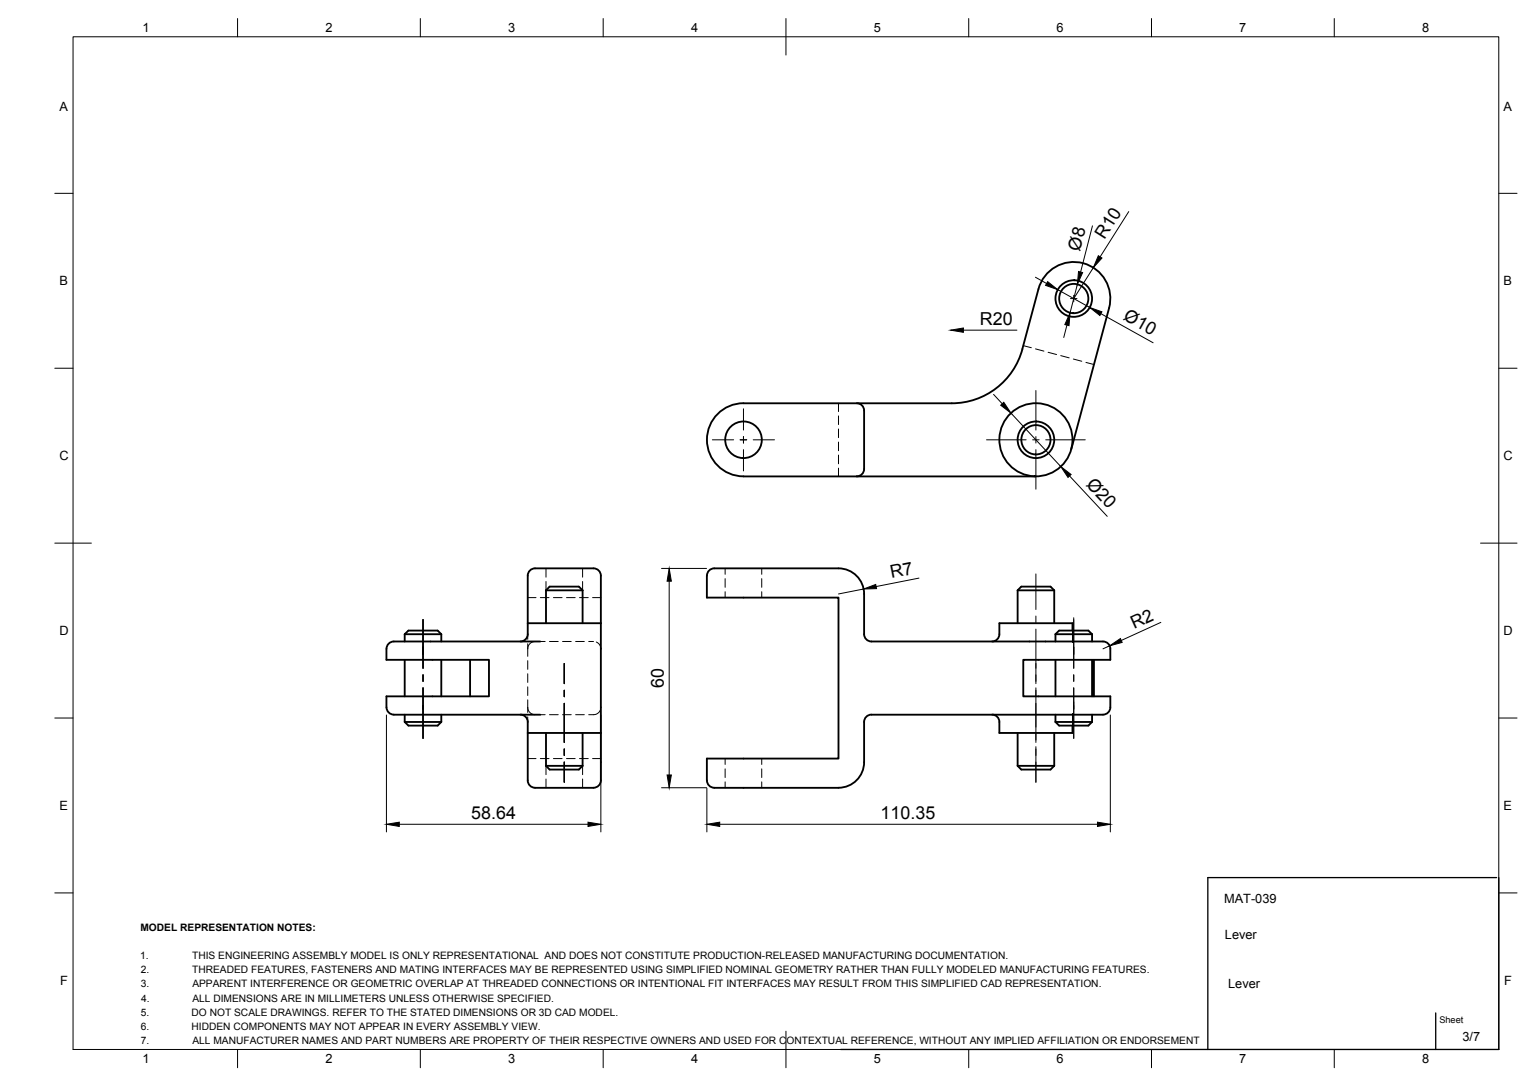
ISO-10303-21;
HEADER;
/* Generated by software containing ST-Developer
 * from STEP Tools, Inc. (www.steptools.com) 
 */

FILE_DESCRIPTION(
/* description */ ('STEP AP214'),
/* implementation_level */ '2;1');

FILE_NAME(
/* name */ 'Lever.step',
/* time_stamp */ '2026-11-14T21:46:24-08:00',
/* author */ (''),
/* organization */ (''),
/* preprocessor_version */ 'ST-DEVELOPER v20.2',
/* originating_system */ 'Autodesk Translation Framework v15.17.0.0',
/* authorisation */ '');

FILE_SCHEMA (('AUTOMOTIVE_DESIGN { 1 0 10303 214 3 1 1 }'));
ENDSEC;

DATA;
#10=MECHANICAL_DESIGN_GEOMETRIC_PRESENTATION_REPRESENTATION('',(#93),#7783);
#11=(
BOUNDED_SURFACE()
B_SPLINE_SURFACE(3,2,((#7242,#7243,#7244),(#7245,#7246,#7247),(#7248,#7249,
#7250),(#7251,#7252,#7253),(#7254,#7255,#7256),(#7257,#7258,#7259),(#7260,
#7261,#7262),(#7263,#7264,#7265),(#7266,#7267,#7268),(#7269,#7270,#7271),
(#7272,#7273,#7274),(#7275,#7276,#7277),(#7278,#7279,#7280),(#7281,#7282,
#7283)),.UNSPECIFIED.,.F.,.F.,.F.)
B_SPLINE_SURFACE_WITH_KNOTS((4,2,2,2,2,2,4),(3,3),(0.00201286221565559,
0.00340012561105001,0.00476544226438698,0.00613075891772395,0.00749607557106092,
0.0102267088777349,0.0129573421844088),(0.,1.00002194674206),
 .UNSPECIFIED.)
GEOMETRIC_REPRESENTATION_ITEM()
RATIONAL_B_SPLINE_SURFACE(((1.,0.706119316799645,1.0000128994471),(1.,0.726784777924549,
1.00001199236801),(1.,0.747777874428932,1.00001107090786),(1.,0.788599708818028,
1.00000927909532),(1.,0.808519289419434,1.00000840475553),(1.,0.845529525851375,
1.0000067802473),(1.,0.862790936611022,1.00000602258384),(1.,0.894561465950779,
1.00000462806462),(1.,0.909105255838781,1.00000398968701),(1.,0.948117278028828,
1.00000227731343),(1.,0.967426794359605,1.00000142975148),(1.,0.993377057003404,
1.00000029070404),(1.,0.999996114407628,1.00000000017055),(1.,1.,1.)))
REPRESENTATION_ITEM('')
SURFACE()
);
#12=(
BOUNDED_SURFACE()
B_SPLINE_SURFACE(3,2,((#7288,#7289,#7290),(#7291,#7292,#7293),(#7294,#7295,
#7296),(#7297,#7298,#7299),(#7300,#7301,#7302),(#7303,#7304,#7305),(#7306,
#7307,#7308),(#7309,#7310,#7311),(#7312,#7313,#7314),(#7315,#7316,#7317),
(#7318,#7319,#7320),(#7321,#7322,#7323),(#7324,#7325,#7326),(#7327,#7328,
#7329)),.UNSPECIFIED.,.F.,.F.,.F.)
B_SPLINE_SURFACE_WITH_KNOTS((4,2,2,2,2,2,4),(3,3),(0.00201286221604104,
0.00340012561105,0.00476544226438698,0.00613075891772395,0.00749607557106092,
0.0102267088777349,0.0129573421844088),(-2.19467416719971E-5,1.00004202921769),
 .UNSPECIFIED.)
GEOMETRIC_REPRESENTATION_ITEM()
RATIONAL_B_SPLINE_SURFACE(((1.00001289944687,0.706106964970707,1.00002470364651),
(1.0000119923678,0.726773294662226,1.00002296650529),(1.00001107090767,
0.747767273503531,1.00002120182301),(1.00000927909516,0.788590823634209,
1.00001777033457),(1.00000840475538,0.808511241458396,1.00001609589217),
(1.00000678024718,0.845523033435795,1.00001298480712),(1.00000602258374,
0.862785169694921,1.00001153381081),(1.00000462806454,0.894557034354464,
1.00000886317619),(1.00000398968694,0.909101435519961,1.00000764062341),
(1.00000227731339,0.948115097390828,1.00000436126801),(1.00000142975146,
0.967425425303272,1.00000273810769),(1.00000029070404,0.993376778640135,
1.00000055672541),(1.00000000017055,0.999996114244353,1.00000000032662),
(1.,1.,1.)))
REPRESENTATION_ITEM('')
SURFACE()
);
#13=(
BOUNDED_SURFACE()
B_SPLINE_SURFACE(3,2,((#7444,#7445,#7446),(#7447,#7448,#7449),(#7450,#7451,
#7452),(#7453,#7454,#7455),(#7456,#7457,#7458),(#7459,#7460,#7461),(#7462,
#7463,#7464),(#7465,#7466,#7467),(#7468,#7469,#7470),(#7471,#7472,#7473),
(#7474,#7475,#7476),(#7477,#7478,#7479),(#7480,#7481,#7482),(#7483,#7484,
#7485)),.UNSPECIFIED.,.F.,.F.,.F.)
B_SPLINE_SURFACE_WITH_KNOTS((4,2,2,2,2,2,4),(3,3),(0.00203480895771304,
0.00340012561105001,0.00476544226438698,0.00613075891772395,0.00749607557106092,
0.0102267088777349,0.0129573421844088),(0.,1.),.UNSPECIFIED.)
GEOMETRIC_REPRESENTATION_ITEM()
RATIONAL_B_SPLINE_SURFACE(((1.,0.707106781186548,1.),(1.,0.727454883115531,
1.),(1.,0.748108881352396,1.),(1.,0.788604348263869,1.),(1.,0.808523491704972,
1.),(1.,0.845532915900626,1.),(1.,0.862793947836832,1.),(1.,0.89456377993233,
1.),(1.,0.909107250638557,1.),(1.,0.948118416660453,1.),(1.,0.967427509219659,
1.),(1.,0.993377202352236,1.),(1.,0.999996114492902,1.),(1.,1.,1.)))
REPRESENTATION_ITEM('')
SURFACE()
);
#14=(
BOUNDED_SURFACE()
B_SPLINE_SURFACE(3,2,((#7492,#7493,#7494),(#7495,#7496,#7497),(#7498,#7499,
#7500),(#7501,#7502,#7503),(#7504,#7505,#7506),(#7507,#7508,#7509),(#7510,
#7511,#7512),(#7513,#7514,#7515),(#7516,#7517,#7518),(#7519,#7520,#7521),
(#7522,#7523,#7524),(#7525,#7526,#7527),(#7528,#7529,#7530),(#7531,#7532,
#7533)),.UNSPECIFIED.,.F.,.F.,.F.)
B_SPLINE_SURFACE_WITH_KNOTS((4,2,2,2,2,2,4),(3,3),(0.00203480895771304,
0.00340012561105001,0.00476544226438698,0.00613075891772395,0.00749607557106092,
0.0102267088777349,0.0129573421844088),(-4.20282077345397E-5,1.),
 .UNSPECIFIED.)
GEOMETRIC_REPRESENTATION_ITEM()
RATIONAL_B_SPLINE_SURFACE(((1.0000246205888,0.707094471409503,1.),(1.00002291012841,
0.727443428532761,1.),(1.00002117395439,0.74809829482011,1.),(1.00001776990754,
0.788595463683529,1.),(1.00001609550537,0.808515444290505,1.),(1.00001298449509,
0.845526423925928,1.),(1.00001153353364,0.862788181312395,1.),(1.0000088629632,
0.894559348636945,1.),(1.0000076404398,0.909103430579154,1.),(1.00000436116321,
0.948116236170593,1.),(1.00000273804189,0.967426140256249,1.),(1.00000055671203,
0.99337692400792,1.),(1.00000000032662,0.999996114329601,1.),(1.,1.,1.)))
REPRESENTATION_ITEM('')
SURFACE()
);
#15=B_SPLINE_CURVE_WITH_KNOTS('',3,(#6784,#6785,#6786,#6787,#6788,#6789,
#6790,#6791,#6792,#6793,#6794,#6795,#6796,#6797,#6798,#6799,#6800,#6801,
#6802,#6803,#6804,#6805,#6806,#6807,#6808,#6809,#6810,#6811,#6812,#6813,
#6814,#6815,#6816,#6817,#6818,#6819,#6820,#6821,#6822,#6823,#6824,#6825,
#6826,#6827,#6828,#6829,#6830,#6831,#6832),.UNSPECIFIED.,.F.,.F.,(4,3,3,
3,3,3,3,3,3,3,3,3,3,3,3,3,4),(0.,0.000463967413666575,0.000954777042109378,
0.00114718345131556,0.00157257184718515,0.0019889538699822,0.00230336685082165,
0.00277738225277823,0.00314514369437031,0.0034731976359017,0.00393142961796289,
0.00434870227875263,0.00465308895983082,0.00471771554155546,0.00539019410311121,
0.00607303876857302,0.00629028738874061),.UNSPECIFIED.);
#16=B_SPLINE_CURVE_WITH_KNOTS('',3,(#6834,#6835,#6836,#6837,#6838,#6839),
 .UNSPECIFIED.,.F.,.F.,(4,2,4),(0.00629028738874061,0.0078707452346593,
0.00945120308057799),.UNSPECIFIED.);
#17=B_SPLINE_CURVE_WITH_KNOTS('',3,(#6843,#6844,#6845,#6846,#6847,#6848),
 .UNSPECIFIED.,.F.,.F.,(4,2,4),(-2.00176139701977E-5,0.00156468827612987,
0.00314939416622993),.UNSPECIFIED.);
#18=B_SPLINE_CURVE_WITH_KNOTS('',3,(#6849,#6850,#6851,#6852,#6853,#6854,
#6855,#6856,#6857,#6858,#6859,#6860,#6861,#6862,#6863,#6864,#6865,#6866,
#6867,#6868,#6869,#6870,#6871,#6872,#6873,#6874,#6875,#6876,#6877,#6878,
#6879,#6880,#6881,#6882,#6883,#6884,#6885,#6886,#6887,#6888,#6889,#6890,
#6891,#6892,#6893,#6894,#6895,#6896,#6897),.UNSPECIFIED.,.F.,.F.,(4,3,3,
3,3,3,3,3,3,3,3,3,3,3,3,3,4),(0.00314939416622993,0.00383486824301925,0.00450997916923667,
0.00472621979976512,0.00479102119555099,0.00520942257342087,0.00551463261653271,
0.00597410411013286,0.0063030454333003,0.0067783430407421,0.00714709927223923,
0.00756460760297828,0.00787987106683548,0.0083064101327715,0.00880180611055996,
0.00926887465145742,0.00945669670037066),.UNSPECIFIED.);
#19=B_SPLINE_CURVE_WITH_KNOTS('',3,(#6902,#6903,#6904,#6905,#6906,#6907,
#6908,#6909,#6910,#6911,#6912,#6913,#6914,#6915,#6916,#6917,#6918,#6919,
#6920,#6921,#6922,#6923,#6924,#6925,#6926,#6927,#6928,#6929,#6930,#6931,
#6932,#6933,#6934,#6935,#6936,#6937,#6938,#6939,#6940,#6941,#6942,#6943,
#6944,#6945,#6946,#6947,#6948,#6949,#6950,#6951,#6952,#6953,#6954,#6955,
#6956,#6957,#6958,#6959,#6960,#6961,#6962,#6963,#6964,#6965,#6966,#6967,
#6968),.UNSPECIFIED.,.F.,.F.,(4,3,3,3,3,3,3,3,3,3,3,3,3,3,3,3,3,3,3,3,3,
3,4),(0.,0.000573434007013873,0.00114686801402775,0.00118140038507225,0.00174268388294295,
0.00230396738081366,0.0023628007701445,0.00306787423031747,0.00347315409373973,
0.00354420115521674,0.0040039106218915,0.0044814901760133,0.00465309204256514,
0.00472560154028899,0.00565974635025426,0.00664141956317292,0.00704595844743703,
0.00708840231043349,0.0077443311007397,0.00826980269550574,0.00881956648446386,
0.00937303729633357,0.00945120308057799),.UNSPECIFIED.);
#20=B_SPLINE_CURVE_WITH_KNOTS('',3,(#6972,#6973,#6974,#6975,#6976,#6977,
#6978,#6979,#6980,#6981,#6982,#6983,#6984,#6985,#6986,#6987,#6988,#6989,
#6990,#6991,#6992,#6993,#6994,#6995,#6996,#6997,#6998,#6999,#7000,#7001,
#7002,#7003,#7004,#7005,#7006,#7007,#7008,#7009,#7010,#7011,#7012,#7013,
#7014,#7015,#7016,#7017,#7018,#7019,#7020,#7021,#7022,#7023,#7024,#7025,
#7026,#7027,#7028,#7029,#7030,#7031,#7032,#7033,#7034,#7035),
 .UNSPECIFIED.,.F.,.F.,(4,3,3,3,3,3,3,3,3,3,3,3,3,3,3,3,3,3,3,3,3,4),(-2.00176139701506E-5,
0.000743071051629322,0.00154611600812219,0.00230505274395684,0.00234916096461506,
0.00239167902346657,0.00338088357647153,0.00432175791491912,0.00471833954320027,
0.00479101813919611,0.0052714217586875,0.00573373183999769,0.00590292883249288,
0.00597414776682822,0.00668110904687163,0.00708751812178548,0.00714649712036357,
0.00770930226572083,0.00827210741107809,0.00830672642201829,0.00888171156119449,
0.0094566967003707),.UNSPECIFIED.);
#21=B_SPLINE_CURVE_WITH_KNOTS('',3,(#7224,#7225,#7226,#7227,#7228,#7229,
#7230,#7231,#7232,#7233,#7234,#7235,#7236,#7237,#7238,#7239),
 .UNSPECIFIED.,.F.,.F.,(4,2,2,2,2,2,2,4),(0.,0.0011867209290651,0.0023734418581302,
0.00356016278719531,0.00474688371626041,0.00712032557439061,0.00830704650345571,
0.00949376743252081),.UNSPECIFIED.);
#22=B_SPLINE_CURVE_WITH_KNOTS('',3,(#7330,#7331,#7332,#7333,#7334,#7335,
#7336,#7337,#7338,#7339,#7340,#7341,#7342,#7343,#7344,#7345),
 .UNSPECIFIED.,.F.,.F.,(4,2,2,2,2,2,2,4),(0.,0.0011867209290651,0.00237344185813019,
0.00356016278719529,0.00474688371626039,0.00712032557439059,0.00830704650345569,
0.00949376743252079),.UNSPECIFIED.);
#23=B_SPLINE_CURVE_WITH_KNOTS('',3,(#7372,#7373,#7374,#7375,#7376,#7377,
#7378,#7379,#7380,#7381,#7382,#7383,#7384,#7385,#7386,#7387,#7388,#7389,
#7390,#7391,#7392,#7393,#7394,#7395,#7396,#7397,#7398,#7399,#7400,#7401,
#7402,#7403,#7404,#7405,#7406,#7407,#7408,#7409,#7410,#7411,#7412,#7413,
#7414,#7415,#7416,#7417,#7418,#7419,#7420,#7421,#7422,#7423,#7424,#7425,
#7426,#7427,#7428,#7429,#7430,#7431,#7432,#7433,#7434,#7435,#7436,#7437,
#7438,#7439,#7440,#7441),.UNSPECIFIED.,.F.,.F.,(4,3,3,3,3,3,3,3,3,3,3,3,
3,3,3,3,3,3,3,3,3,3,3,4),(-2.20338883785527E-5,0.000642558597019686,0.00116395721593939,
0.00201707586197036,0.00234994832025733,0.00244440929736401,0.00317109830627835,
0.00387836420487405,0.00455999932782322,0.00472193052889321,0.00487208598317901,
0.00547292850863629,0.00607377103409357,0.00663117903387144,0.00709391273752908,
0.00724862880926105,0.00759056213579682,0.00791199062197989,0.0082104406191189,
0.00827990384184702,0.00838782827049795,0.00882409089832456,0.00926054923459336,
0.00946589494616496),.UNSPECIFIED.);
#24=B_SPLINE_CURVE_WITH_KNOTS('',3,(#7534,#7535,#7536,#7537,#7538,#7539,
#7540,#7541,#7542,#7543,#7544,#7545,#7546,#7547,#7548,#7549,#7550,#7551,
#7552,#7553,#7554,#7555,#7556,#7557,#7558,#7559,#7560,#7561,#7562,#7563,
#7564,#7565,#7566,#7567,#7568,#7569,#7570,#7571,#7572,#7573,#7574,#7575,
#7576,#7577,#7578,#7579,#7580,#7581,#7582,#7583,#7584,#7585,#7586,#7587,
#7588,#7589,#7590,#7591,#7592,#7593,#7594,#7595,#7596,#7597,#7598,#7599,
#7600,#7601,#7602,#7603),.UNSPECIFIED.,.F.,.F.,(4,3,3,3,3,3,3,3,3,3,3,3,
3,3,3,3,3,3,3,3,3,3,3,4),(-2.20338883785244E-5,0.000642558597506865,0.00116395721593941,
0.00201707586185835,0.00234994832025735,0.00244440929736402,0.00317109830623264,
0.00387836420476937,0.0045599993276549,0.00472193052889323,0.00487208598317904,
0.00547292850863634,0.00607377103409363,0.00663117903387409,0.00709391273752911,
0.00724862880926107,0.00759056213580112,0.00791199062198886,0.00821044061913349,
0.00827990384184705,0.00838782827049793,0.00882409089835773,0.00926054923468115,
0.00946589494616499),.UNSPECIFIED.);
#79=SHAPE_REPRESENTATION_RELATIONSHIP('SRR','None',#7824,#86);
#86=ADVANCED_BREP_SHAPE_REPRESENTATION('',(#100),#7780);
#93=STYLED_ITEM('',(#7868),#100);
#100=MANIFOLD_SOLID_BREP('Body1',#4168);
#104=CONICAL_SURFACE('',#4479,3.99999999999998,0.785398163397453);
#105=CONICAL_SURFACE('',#4482,3.99999999999998,0.785398163397454);
#106=CONICAL_SURFACE('',#4485,5.,0.785398163397443);
#107=CONICAL_SURFACE('',#4489,5.,0.785398163397443);
#141=FACE_BOUND('',#1509,.T.);
#142=FACE_BOUND('',#1516,.T.);
#143=FACE_BOUND('',#1520,.T.);
#144=FACE_BOUND('',#1523,.T.);
#145=FACE_BOUND('',#1526,.T.);
#146=FACE_BOUND('',#1528,.T.);
#147=FACE_BOUND('',#1530,.T.);
#148=FACE_BOUND('',#1533,.T.);
#149=FACE_BOUND('',#1535,.T.);
#150=FACE_BOUND('',#1538,.T.);
#248=PLANE('',#4536);
#249=PLANE('',#4539);
#250=PLANE('',#4540);
#251=PLANE('',#4544);
#252=PLANE('',#4549);
#253=PLANE('',#4554);
#254=PLANE('',#4557);
#255=PLANE('',#4558);
#256=PLANE('',#4559);
#257=PLANE('',#4560);
#258=PLANE('',#4561);
#259=PLANE('',#4562);
#260=PLANE('',#4563);
#261=PLANE('',#4566);
#262=PLANE('',#4571);
#263=PLANE('',#4572);
#264=PLANE('',#4573);
#265=PLANE('',#4574);
#266=PLANE('',#4642);
#267=PLANE('',#4643);
#268=PLANE('',#4644);
#269=PLANE('',#4645);
#522=LINE('',#6674,#881);
#523=LINE('',#6680,#882);
#524=LINE('',#6688,#883);
#525=LINE('',#6696,#884);
#526=LINE('',#6701,#885);
#527=LINE('',#6704,#886);
#528=LINE('',#6710,#887);
#529=LINE('',#6715,#888);
#530=LINE('',#6718,#889);
#531=LINE('',#6753,#890);
#532=LINE('',#6757,#891);
#533=LINE('',#6760,#892);
#534=LINE('',#6765,#893);
#535=LINE('',#6772,#894);
#536=LINE('',#6775,#895);
#537=LINE('',#6780,#896);
#538=LINE('',#6841,#897);
#539=LINE('',#6899,#898);
#540=LINE('',#6970,#899);
#541=LINE('',#7039,#900);
#542=LINE('',#7043,#901);
#543=LINE('',#7047,#902);
#544=LINE('',#7049,#903);
#545=LINE('',#7050,#904);
#546=LINE('',#7052,#905);
#547=LINE('',#7053,#906);
#548=LINE('',#7055,#907);
#549=LINE('',#7057,#908);
#550=LINE('',#7058,#909);
#551=LINE('',#7062,#910);
#552=LINE('',#7063,#911);
#553=LINE('',#7065,#912);
#554=LINE('',#7067,#913);
#555=LINE('',#7068,#914);
#556=LINE('',#7069,#915);
#557=LINE('',#7073,#916);
#558=LINE('',#7078,#917);
#559=LINE('',#7080,#918);
#560=LINE('',#7084,#919);
#561=LINE('',#7087,#920);
#562=LINE('',#7089,#921);
#563=LINE('',#7093,#922);
#564=LINE('',#7097,#923);
#565=LINE('',#7099,#924);
#566=LINE('',#7101,#925);
#567=LINE('',#7103,#926);
#568=LINE('',#7104,#927);
#569=LINE('',#7109,#928);
#570=LINE('',#7111,#929);
#571=LINE('',#7113,#930);
#572=LINE('',#7115,#931);
#573=LINE('',#7117,#932);
#574=LINE('',#7119,#933);
#575=LINE('',#7121,#934);
#576=LINE('',#7125,#935);
#577=LINE('',#7128,#936);
#578=LINE('',#7130,#937);
#579=LINE('',#7133,#938);
#580=LINE('',#7137,#939);
#581=LINE('',#7138,#940);
#582=LINE('',#7139,#941);
#583=LINE('',#7143,#942);
#584=LINE('',#7144,#943);
#585=LINE('',#7147,#944);
#586=LINE('',#7148,#945);
#587=LINE('',#7153,#946);
#588=LINE('',#7155,#947);
#589=LINE('',#7157,#948);
#590=LINE('',#7158,#949);
#591=LINE('',#7162,#950);
#592=LINE('',#7164,#951);
#593=LINE('',#7168,#952);
#594=LINE('',#7170,#953);
#595=LINE('',#7172,#954);
#596=LINE('',#7179,#955);
#597=LINE('',#7181,#956);
#598=LINE('',#7182,#957);
#599=LINE('',#7191,#958);
#600=LINE('',#7193,#959);
#601=LINE('',#7195,#960);
#602=LINE('',#7196,#961);
#881=VECTOR('',#5409,3.99999999999998);
#882=VECTOR('',#5416,3.99999999999998);
#883=VECTOR('',#5425,5.);
#884=VECTOR('',#5434,5.);
#885=VECTOR('',#5441,5.);
#886=VECTOR('',#5444,5.);
#887=VECTOR('',#5451,5.);
#888=VECTOR('',#5458,5.);
#889=VECTOR('',#5461,5.);
#890=VECTOR('',#5500,5.);
#891=VECTOR('',#5505,1000.);
#892=VECTOR('',#5508,1000.);
#893=VECTOR('',#5513,5.);
#894=VECTOR('',#5520,1000.);
#895=VECTOR('',#5523,1000.);
#896=VECTOR('',#5528,10.);
#897=VECTOR('',#5531,1000.);
#898=VECTOR('',#5532,10.);
#899=VECTOR('',#5535,1000.);
#900=VECTOR('',#5540,1000.);
#901=VECTOR('',#5543,1000.);
#902=VECTOR('',#5546,1000.);
#903=VECTOR('',#5547,1000.);
#904=VECTOR('',#5548,1000.);
#905=VECTOR('',#5551,1000.);
#906=VECTOR('',#5552,1000.);
#907=VECTOR('',#5553,1000.);
#908=VECTOR('',#5554,1000.);
#909=VECTOR('',#5555,1000.);
#910=VECTOR('',#5558,1000.);
#911=VECTOR('',#5559,1000.);
#912=VECTOR('',#5560,1000.);
#913=VECTOR('',#5561,1000.);
#914=VECTOR('',#5562,1000.);
#915=VECTOR('',#5563,1000.);
#916=VECTOR('',#5566,1000.);
#917=VECTOR('',#5573,1000.);
#918=VECTOR('',#5574,1000.);
#919=VECTOR('',#5577,1000.);
#920=VECTOR('',#5580,1000.);
#921=VECTOR('',#5581,1000.);
#922=VECTOR('',#5584,1000.);
#923=VECTOR('',#5587,1000.);
#924=VECTOR('',#5588,1000.);
#925=VECTOR('',#5589,1000.);
#926=VECTOR('',#5590,1000.);
#927=VECTOR('',#5591,1000.);
#928=VECTOR('',#5596,1000.);
#929=VECTOR('',#5597,1000.);
#930=VECTOR('',#5598,1000.);
#931=VECTOR('',#5599,1000.);
#932=VECTOR('',#5600,1000.);
#933=VECTOR('',#5601,1000.);
#934=VECTOR('',#5602,1000.);
#935=VECTOR('',#5605,1000.);
#936=VECTOR('',#5608,1000.);
#937=VECTOR('',#5609,1000.);
#938=VECTOR('',#5612,1000.);
#939=VECTOR('',#5615,1000.);
#940=VECTOR('',#5616,1000.);
#941=VECTOR('',#5617,1000.);
#942=VECTOR('',#5624,1000.);
#943=VECTOR('',#5625,1000.);
#944=VECTOR('',#5630,1000.);
#945=VECTOR('',#5631,1000.);
#946=VECTOR('',#5636,1000.);
#947=VECTOR('',#5637,1000.);
#948=VECTOR('',#5638,1000.);
#949=VECTOR('',#5639,1000.);
#950=VECTOR('',#5644,1000.);
#951=VECTOR('',#5645,1000.);
#952=VECTOR('',#5648,1000.);
#953=VECTOR('',#5649,1000.);
#954=VECTOR('',#5650,1000.);
#955=VECTOR('',#5657,1000.);
#956=VECTOR('',#5658,1000.);
#957=VECTOR('',#5659,1000.);
#958=VECTOR('',#5672,1000.);
#959=VECTOR('',#5673,1000.);
#960=VECTOR('',#5674,1000.);
#961=VECTOR('',#5675,1000.);
#1045=CYLINDRICAL_SURFACE('',#4493,5.);
#1046=CYLINDRICAL_SURFACE('',#4495,5.);
#1047=CYLINDRICAL_SURFACE('',#4497,5.);
#1048=CYLINDRICAL_SURFACE('',#4500,5.);
#1049=CYLINDRICAL_SURFACE('',#4502,5.);
#1050=CYLINDRICAL_SURFACE('',#4520,5.);
#1051=CYLINDRICAL_SURFACE('',#4523,10.);
#1052=CYLINDRICAL_SURFACE('',#4525,5.);
#1053=CYLINDRICAL_SURFACE('',#4528,10.);
#1054=CYLINDRICAL_SURFACE('',#4531,10.);
#1055=CYLINDRICAL_SURFACE('',#4541,20.);
#1056=CYLINDRICAL_SURFACE('',#4555,10.);
#1057=CYLINDRICAL_SURFACE('',#4568,10.);
#1058=CYLINDRICAL_SURFACE('',#4575,7.);
#1059=CYLINDRICAL_SURFACE('',#4578,7.);
#1060=CYLINDRICAL_SURFACE('',#4581,2.);
#1061=CYLINDRICAL_SURFACE('',#4583,2.);
#1062=CYLINDRICAL_SURFACE('',#4589,2.);
#1063=CYLINDRICAL_SURFACE('',#4591,2.);
#1064=CYLINDRICAL_SURFACE('',#4594,2.);
#1065=CYLINDRICAL_SURFACE('',#4600,2.);
#1066=CYLINDRICAL_SURFACE('',#4601,2.);
#1067=CYLINDRICAL_SURFACE('',#4605,2.);
#1068=CYLINDRICAL_SURFACE('',#4609,2.);
#1069=CYLINDRICAL_SURFACE('',#4613,2.);
#1070=CYLINDRICAL_SURFACE('',#4615,2.);
#1071=CYLINDRICAL_SURFACE('',#4621,2.);
#1072=CYLINDRICAL_SURFACE('',#4623,2.);
#1073=CYLINDRICAL_SURFACE('',#4625,2.);
#1074=CYLINDRICAL_SURFACE('',#4632,2.);
#1075=CYLINDRICAL_SURFACE('',#4633,2.);
#1076=CYLINDRICAL_SURFACE('',#4640,2.);
#1077=CYLINDRICAL_SURFACE('',#4641,2.);
#1219=FACE_OUTER_BOUND('',#1491,.T.);
#1220=FACE_OUTER_BOUND('',#1492,.T.);
#1221=FACE_OUTER_BOUND('',#1493,.T.);
#1222=FACE_OUTER_BOUND('',#1494,.T.);
#1223=FACE_OUTER_BOUND('',#1495,.T.);
#1224=FACE_OUTER_BOUND('',#1496,.T.);
#1225=FACE_OUTER_BOUND('',#1497,.T.);
#1226=FACE_OUTER_BOUND('',#1498,.T.);
#1227=FACE_OUTER_BOUND('',#1499,.T.);
#1228=FACE_OUTER_BOUND('',#1500,.T.);
#1229=FACE_OUTER_BOUND('',#1501,.T.);
#1230=FACE_OUTER_BOUND('',#1502,.T.);
#1231=FACE_OUTER_BOUND('',#1503,.T.);
#1232=FACE_OUTER_BOUND('',#1504,.T.);
#1233=FACE_OUTER_BOUND('',#1505,.T.);
#1234=FACE_OUTER_BOUND('',#1506,.T.);
#1235=FACE_OUTER_BOUND('',#1507,.T.);
#1236=FACE_OUTER_BOUND('',#1508,.T.);
#1237=FACE_OUTER_BOUND('',#1510,.T.);
#1238=FACE_OUTER_BOUND('',#1511,.T.);
#1239=FACE_OUTER_BOUND('',#1512,.T.);
#1240=FACE_OUTER_BOUND('',#1513,.T.);
#1241=FACE_OUTER_BOUND('',#1514,.T.);
#1242=FACE_OUTER_BOUND('',#1515,.T.);
#1243=FACE_OUTER_BOUND('',#1517,.T.);
#1244=FACE_OUTER_BOUND('',#1518,.T.);
#1245=FACE_OUTER_BOUND('',#1519,.T.);
#1246=FACE_OUTER_BOUND('',#1521,.T.);
#1247=FACE_OUTER_BOUND('',#1522,.T.);
#1248=FACE_OUTER_BOUND('',#1524,.T.);
#1249=FACE_OUTER_BOUND('',#1525,.T.);
#1250=FACE_OUTER_BOUND('',#1527,.T.);
#1251=FACE_OUTER_BOUND('',#1529,.T.);
#1252=FACE_OUTER_BOUND('',#1531,.T.);
#1253=FACE_OUTER_BOUND('',#1532,.T.);
#1254=FACE_OUTER_BOUND('',#1534,.T.);
#1255=FACE_OUTER_BOUND('',#1536,.T.);
#1256=FACE_OUTER_BOUND('',#1537,.T.);
#1257=FACE_OUTER_BOUND('',#1539,.T.);
#1258=FACE_OUTER_BOUND('',#1540,.T.);
#1259=FACE_OUTER_BOUND('',#1541,.T.);
#1260=FACE_OUTER_BOUND('',#1542,.T.);
#1261=FACE_OUTER_BOUND('',#1543,.T.);
#1262=FACE_OUTER_BOUND('',#1544,.T.);
#1263=FACE_OUTER_BOUND('',#1545,.T.);
#1264=FACE_OUTER_BOUND('',#1546,.T.);
#1265=FACE_OUTER_BOUND('',#1547,.T.);
#1266=FACE_OUTER_BOUND('',#1548,.T.);
#1267=FACE_OUTER_BOUND('',#1549,.T.);
#1268=FACE_OUTER_BOUND('',#1550,.T.);
#1269=FACE_OUTER_BOUND('',#1551,.T.);
#1270=FACE_OUTER_BOUND('',#1552,.T.);
#1271=FACE_OUTER_BOUND('',#1553,.T.);
#1272=FACE_OUTER_BOUND('',#1554,.T.);
#1273=FACE_OUTER_BOUND('',#1555,.T.);
#1274=FACE_OUTER_BOUND('',#1556,.T.);
#1275=FACE_OUTER_BOUND('',#1557,.T.);
#1276=FACE_OUTER_BOUND('',#1558,.T.);
#1277=FACE_OUTER_BOUND('',#1559,.T.);
#1278=FACE_OUTER_BOUND('',#1560,.T.);
#1279=FACE_OUTER_BOUND('',#1561,.T.);
#1280=FACE_OUTER_BOUND('',#1562,.T.);
#1281=FACE_OUTER_BOUND('',#1563,.T.);
#1282=FACE_OUTER_BOUND('',#1564,.T.);
#1283=FACE_OUTER_BOUND('',#1565,.T.);
#1284=FACE_OUTER_BOUND('',#1566,.T.);
#1285=FACE_OUTER_BOUND('',#1567,.T.);
#1286=FACE_OUTER_BOUND('',#1568,.T.);
#1287=FACE_OUTER_BOUND('',#1569,.T.);
#1288=FACE_OUTER_BOUND('',#1570,.T.);
#1289=FACE_OUTER_BOUND('',#1571,.T.);
#1290=FACE_OUTER_BOUND('',#1572,.T.);
#1291=FACE_OUTER_BOUND('',#1573,.T.);
#1292=FACE_OUTER_BOUND('',#1574,.T.);
#1293=FACE_OUTER_BOUND('',#1575,.T.);
#1294=FACE_OUTER_BOUND('',#1576,.T.);
#1295=FACE_OUTER_BOUND('',#1577,.T.);
#1296=FACE_OUTER_BOUND('',#1578,.T.);
#1297=FACE_OUTER_BOUND('',#1579,.T.);
#1491=EDGE_LOOP('',(#3402,#3403,#3404,#3405));
#1492=EDGE_LOOP('',(#3406,#3407,#3408,#3409));
#1493=EDGE_LOOP('',(#3410,#3411,#3412,#3413,#3414));
#1494=EDGE_LOOP('',(#3415,#3416,#3417,#3418,#3419));
#1495=EDGE_LOOP('',(#3420,#3421,#3422,#3423));
#1496=EDGE_LOOP('',(#3424,#3425,#3426,#3427,#3428));
#1497=EDGE_LOOP('',(#3429,#3430,#3431,#3432));
#1498=EDGE_LOOP('',(#3433,#3434,#3435,#3436));
#1499=EDGE_LOOP('',(#3437,#3438,#3439,#3440,#3441));
#1500=EDGE_LOOP('',(#3442,#3443,#3444,#3445));
#1501=EDGE_LOOP('',(#3446,#3447,#3448,#3449,#3450));
#1502=EDGE_LOOP('',(#3451,#3452,#3453,#3454));
#1503=EDGE_LOOP('',(#3455,#3456,#3457,#3458));
#1504=EDGE_LOOP('',(#3459,#3460,#3461,#3462));
#1505=EDGE_LOOP('',(#3463,#3464,#3465,#3466));
#1506=EDGE_LOOP('',(#3467,#3468,#3469,#3470));
#1507=EDGE_LOOP('',(#3471,#3472,#3473,#3474,#3475,#3476,#3477,#3478,#3479,
#3480,#3481,#3482,#3483,#3484,#3485,#3486,#3487,#3488));
#1508=EDGE_LOOP('',(#3489,#3490,#3491,#3492,#3493,#3494,#3495,#3496));
#1509=EDGE_LOOP('',(#3497));
#1510=EDGE_LOOP('',(#3498,#3499,#3500,#3501,#3502,#3503,#3504,#3505));
#1511=EDGE_LOOP('',(#3506,#3507,#3508,#3509,#3510,#3511,#3512,#3513));
#1512=EDGE_LOOP('',(#3514,#3515,#3516,#3517));
#1513=EDGE_LOOP('',(#3518,#3519,#3520,#3521,#3522,#3523,#3524,#3525,#3526,
#3527,#3528,#3529,#3530,#3531,#3532,#3533));
#1514=EDGE_LOOP('',(#3534,#3535,#3536,#3537,#3538,#3539,#3540,#3541,#3542,
#3543,#3544,#3545,#3546,#3547,#3548,#3549));
#1515=EDGE_LOOP('',(#3550,#3551,#3552,#3553));
#1516=EDGE_LOOP('',(#3554));
#1517=EDGE_LOOP('',(#3555,#3556,#3557,#3558));
#1518=EDGE_LOOP('',(#3559,#3560,#3561,#3562));
#1519=EDGE_LOOP('',(#3563,#3564,#3565,#3566));
#1520=EDGE_LOOP('',(#3567));
#1521=EDGE_LOOP('',(#3568,#3569,#3570,#3571));
#1522=EDGE_LOOP('',(#3572,#3573,#3574,#3575));
#1523=EDGE_LOOP('',(#3576));
#1524=EDGE_LOOP('',(#3577,#3578,#3579,#3580));
#1525=EDGE_LOOP('',(#3581));
#1526=EDGE_LOOP('',(#3582));
#1527=EDGE_LOOP('',(#3583,#3584,#3585,#3586,#3587,#3588,#3589,#3590));
#1528=EDGE_LOOP('',(#3591));
#1529=EDGE_LOOP('',(#3592,#3593,#3594,#3595));
#1530=EDGE_LOOP('',(#3596));
#1531=EDGE_LOOP('',(#3597,#3598,#3599,#3600));
#1532=EDGE_LOOP('',(#3601,#3602,#3603,#3604));
#1533=EDGE_LOOP('',(#3605));
#1534=EDGE_LOOP('',(#3606,#3607,#3608,#3609));
#1535=EDGE_LOOP('',(#3610));
#1536=EDGE_LOOP('',(#3611,#3612,#3613,#3614));
#1537=EDGE_LOOP('',(#3615));
#1538=EDGE_LOOP('',(#3616));
#1539=EDGE_LOOP('',(#3617,#3618,#3619,#3620));
#1540=EDGE_LOOP('',(#3621,#3622,#3623,#3624));
#1541=EDGE_LOOP('',(#3625,#3626,#3627,#3628));
#1542=EDGE_LOOP('',(#3629,#3630,#3631,#3632));
#1543=EDGE_LOOP('',(#3633,#3634,#3635,#3636));
#1544=EDGE_LOOP('',(#3637,#3638,#3639,#3640));
#1545=EDGE_LOOP('',(#3641,#3642,#3643,#3644));
#1546=EDGE_LOOP('',(#3645,#3646,#3647,#3648));
#1547=EDGE_LOOP('',(#3649,#3650,#3651,#3652));
#1548=EDGE_LOOP('',(#3653,#3654,#3655,#3656));
#1549=EDGE_LOOP('',(#3657,#3658,#3659,#3660));
#1550=EDGE_LOOP('',(#3661,#3662,#3663,#3664));
#1551=EDGE_LOOP('',(#3665,#3666,#3667,#3668));
#1552=EDGE_LOOP('',(#3669,#3670,#3671));
#1553=EDGE_LOOP('',(#3672,#3673,#3674,#3675));
#1554=EDGE_LOOP('',(#3676,#3677,#3678,#3679));
#1555=EDGE_LOOP('',(#3680,#3681,#3682,#3683));
#1556=EDGE_LOOP('',(#3684,#3685,#3686,#3687));
#1557=EDGE_LOOP('',(#3688,#3689,#3690,#3691));
#1558=EDGE_LOOP('',(#3692,#3693,#3694,#3695));
#1559=EDGE_LOOP('',(#3696,#3697,#3698,#3699));
#1560=EDGE_LOOP('',(#3700,#3701,#3702,#3703));
#1561=EDGE_LOOP('',(#3704,#3705,#3706,#3707));
#1562=EDGE_LOOP('',(#3708,#3709,#3710,#3711));
#1563=EDGE_LOOP('',(#3712,#3713,#3714,#3715));
#1564=EDGE_LOOP('',(#3716,#3717,#3718,#3719));
#1565=EDGE_LOOP('',(#3720,#3721,#3722,#3723));
#1566=EDGE_LOOP('',(#3724,#3725,#3726,#3727));
#1567=EDGE_LOOP('',(#3728,#3729,#3730,#3731));
#1568=EDGE_LOOP('',(#3732,#3733,#3734,#3735));
#1569=EDGE_LOOP('',(#3736,#3737,#3738,#3739));
#1570=EDGE_LOOP('',(#3740,#3741,#3742));
#1571=EDGE_LOOP('',(#3743,#3744,#3745,#3746));
#1572=EDGE_LOOP('',(#3747,#3748,#3749,#3750,#3751));
#1573=EDGE_LOOP('',(#3752,#3753,#3754,#3755));
#1574=EDGE_LOOP('',(#3756,#3757,#3758,#3759));
#1575=EDGE_LOOP('',(#3760,#3761,#3762,#3763));
#1576=EDGE_LOOP('',(#3764));
#1577=EDGE_LOOP('',(#3765));
#1578=EDGE_LOOP('',(#3766));
#1579=EDGE_LOOP('',(#3767));
#1708=CIRCLE('',#4480,5.);
#1709=CIRCLE('',#4481,3.99999999999998);
#1710=CIRCLE('',#4483,5.);
#1711=CIRCLE('',#4484,3.99999999999998);
#1712=CIRCLE('',#4486,5.);
#1713=CIRCLE('',#4487,5.);
#1714=CIRCLE('',#4488,3.99999999999999);
#1715=CIRCLE('',#4490,5.);
#1716=CIRCLE('',#4491,5.);
#1717=CIRCLE('',#4492,3.99999999999999);
#1718=CIRCLE('',#4494,5.);
#1719=CIRCLE('',#4496,5.);
#1720=CIRCLE('',#4498,5.);
#1721=CIRCLE('',#4499,5.);
#1722=CIRCLE('',#4501,5.);
#1723=CIRCLE('',#4503,5.);
#1724=CIRCLE('',#4505,10.);
#1725=CIRCLE('',#4506,2.);
#1726=CIRCLE('',#4507,8.);
#1727=CIRCLE('',#4508,2.);
#1728=CIRCLE('',#4510,10.);
#1729=CIRCLE('',#4511,2.);
#1730=CIRCLE('',#4512,12.);
#1731=CIRCLE('',#4513,2.);
#1732=CIRCLE('',#4514,10.);
#1733=CIRCLE('',#4516,10.);
#1734=CIRCLE('',#4517,2.);
#1735=CIRCLE('',#4518,8.00000000000001);
#1736=CIRCLE('',#4519,2.);
#1737=CIRCLE('',#4521,5.);
#1738=CIRCLE('',#4522,5.);
#1739=CIRCLE('',#4524,10.);
#1740=CIRCLE('',#4526,5.);
#1741=CIRCLE('',#4527,5.);
#1742=CIRCLE('',#4529,10.);
#1743=CIRCLE('',#4530,10.);
#1744=CIRCLE('',#4532,10.);
#1745=CIRCLE('',#4533,10.);
#1746=CIRCLE('',#4534,10.);
#1747=CIRCLE('',#4535,10.);
#1748=CIRCLE('',#4537,8.);
#1749=CIRCLE('',#4538,22.);
#1750=CIRCLE('',#4542,20.);
#1751=CIRCLE('',#4543,20.);
#1752=CIRCLE('',#4545,5.);
#1753=CIRCLE('',#4546,4.);
#1754=CIRCLE('',#4547,4.);
#1755=CIRCLE('',#4548,5.);
#1756=CIRCLE('',#4550,5.);
#1757=CIRCLE('',#4551,5.);
#1758=CIRCLE('',#4552,4.);
#1759=CIRCLE('',#4553,4.);
#1760=CIRCLE('',#4556,10.);
#1761=CIRCLE('',#4564,12.);
#1762=CIRCLE('',#4565,22.);
#1763=CIRCLE('',#4567,8.00000000000001);
#1764=CIRCLE('',#4569,10.);
#1765=CIRCLE('',#4570,10.);
#1766=CIRCLE('',#4576,7.);
#1767=CIRCLE('',#4577,7.);
#1768=CIRCLE('',#4579,7.);
#1769=CIRCLE('',#4580,7.);
#1770=CIRCLE('',#4582,2.);
#1771=CIRCLE('',#4584,2.);
#1772=CIRCLE('',#4586,2.);
#1773=CIRCLE('',#4588,2.);
#1774=CIRCLE('',#4590,2.);
#1775=CIRCLE('',#4592,2.);
#1776=CIRCLE('',#4593,2.);
#1777=CIRCLE('',#4595,2.);
#1778=CIRCLE('',#4597,2.);
#1779=CIRCLE('',#4599,2.);
#1780=CIRCLE('',#4602,2.);
#1781=CIRCLE('',#4604,2.);
#1782=CIRCLE('',#4606,2.);
#1783=CIRCLE('',#4608,2.);
#1784=CIRCLE('',#4611,2.);
#1785=CIRCLE('',#4612,2.);
#1786=CIRCLE('',#4614,2.);
#1787=CIRCLE('',#4616,2.);
#1788=CIRCLE('',#4618,2.);
#1789=CIRCLE('',#4620,2.);
#1790=CIRCLE('',#4622,2.);
#1791=CIRCLE('',#4624,2.);
#1792=CIRCLE('',#4626,2.);
#1793=CIRCLE('',#4627,2.);
#1794=CIRCLE('',#4629,2.);
#1795=CIRCLE('',#4631,2.);
#1796=CIRCLE('',#4634,2.);
#1797=CIRCLE('',#4635,2.);
#1798=CIRCLE('',#4637,2.);
#1799=CIRCLE('',#4639,2.);
#2032=VERTEX_POINT('',#6671);
#2033=VERTEX_POINT('',#6673);
#2034=VERTEX_POINT('',#6677);
#2035=VERTEX_POINT('',#6679);
#2036=VERTEX_POINT('',#6683);
#2037=VERTEX_POINT('',#6684);
#2038=VERTEX_POINT('',#6687);
#2039=VERTEX_POINT('',#6691);
#2040=VERTEX_POINT('',#6692);
#2041=VERTEX_POINT('',#6695);
#2042=VERTEX_POINT('',#6699);
#2043=VERTEX_POINT('',#6703);
#2044=VERTEX_POINT('',#6707);
#2045=VERTEX_POINT('',#6709);
#2046=VERTEX_POINT('',#6713);
#2047=VERTEX_POINT('',#6717);
#2048=VERTEX_POINT('',#6721);
#2049=VERTEX_POINT('',#6722);
#2050=VERTEX_POINT('',#6724);
#2051=VERTEX_POINT('',#6726);
#2052=VERTEX_POINT('',#6730);
#2053=VERTEX_POINT('',#6731);
#2054=VERTEX_POINT('',#6733);
#2055=VERTEX_POINT('',#6735);
#2056=VERTEX_POINT('',#6737);
#2057=VERTEX_POINT('',#6741);
#2058=VERTEX_POINT('',#6742);
#2059=VERTEX_POINT('',#6744);
#2060=VERTEX_POINT('',#6746);
#2061=VERTEX_POINT('',#6750);
#2062=VERTEX_POINT('',#6752);
#2063=VERTEX_POINT('',#6756);
#2064=VERTEX_POINT('',#6758);
#2065=VERTEX_POINT('',#6762);
#2066=VERTEX_POINT('',#6764);
#2067=VERTEX_POINT('',#6768);
#2068=VERTEX_POINT('',#6769);
#2069=VERTEX_POINT('',#6771);
#2070=VERTEX_POINT('',#6773);
#2071=VERTEX_POINT('',#6777);
#2072=VERTEX_POINT('',#6779);
#2073=VERTEX_POINT('',#6781);
#2074=VERTEX_POINT('',#6783);
#2075=VERTEX_POINT('',#6833);
#2076=VERTEX_POINT('',#6840);
#2077=VERTEX_POINT('',#6842);
#2078=VERTEX_POINT('',#6898);
#2079=VERTEX_POINT('',#6901);
#2080=VERTEX_POINT('',#6969);
#2081=VERTEX_POINT('',#6971);
#2082=VERTEX_POINT('',#7038);
#2083=VERTEX_POINT('',#7040);
#2084=VERTEX_POINT('',#7042);
#2085=VERTEX_POINT('',#7044);
#2086=VERTEX_POINT('',#7046);
#2087=VERTEX_POINT('',#7048);
#2088=VERTEX_POINT('',#7054);
#2089=VERTEX_POINT('',#7056);
#2090=VERTEX_POINT('',#7060);
#2091=VERTEX_POINT('',#7061);
#2092=VERTEX_POINT('',#7064);
#2093=VERTEX_POINT('',#7066);
#2094=VERTEX_POINT('',#7071);
#2095=VERTEX_POINT('',#7072);
#2096=VERTEX_POINT('',#7077);
#2097=VERTEX_POINT('',#7079);
#2098=VERTEX_POINT('',#7081);
#2099=VERTEX_POINT('',#7083);
#2100=VERTEX_POINT('',#7085);
#2101=VERTEX_POINT('',#7088);
#2102=VERTEX_POINT('',#7090);
#2103=VERTEX_POINT('',#7092);
#2104=VERTEX_POINT('',#7094);
#2105=VERTEX_POINT('',#7096);
#2106=VERTEX_POINT('',#7098);
#2107=VERTEX_POINT('',#7100);
#2108=VERTEX_POINT('',#7102);
#2109=VERTEX_POINT('',#7106);
#2110=VERTEX_POINT('',#7107);
#2111=VERTEX_POINT('',#7110);
#2112=VERTEX_POINT('',#7112);
#2113=VERTEX_POINT('',#7114);
#2114=VERTEX_POINT('',#7116);
#2115=VERTEX_POINT('',#7118);
#2116=VERTEX_POINT('',#7120);
#2117=VERTEX_POINT('',#7122);
#2118=VERTEX_POINT('',#7124);
#2119=VERTEX_POINT('',#7126);
#2120=VERTEX_POINT('',#7129);
#2121=VERTEX_POINT('',#7131);
#2122=VERTEX_POINT('',#7135);
#2123=VERTEX_POINT('',#7136);
#2124=VERTEX_POINT('',#7151);
#2125=VERTEX_POINT('',#7152);
#2126=VERTEX_POINT('',#7154);
#2127=VERTEX_POINT('',#7156);
#2128=VERTEX_POINT('',#7161);
#2129=VERTEX_POINT('',#7163);
#2130=VERTEX_POINT('',#7165);
#2131=VERTEX_POINT('',#7167);
#2132=VERTEX_POINT('',#7169);
#2133=VERTEX_POINT('',#7171);
#2134=VERTEX_POINT('',#7175);
#2135=VERTEX_POINT('',#7176);
#2136=VERTEX_POINT('',#7178);
#2137=VERTEX_POINT('',#7180);
#2138=VERTEX_POINT('',#7189);
#2139=VERTEX_POINT('',#7190);
#2140=VERTEX_POINT('',#7192);
#2141=VERTEX_POINT('',#7194);
#2508=EDGE_CURVE('',#2032,#2032,#1708,.T.);
#2509=EDGE_CURVE('',#2032,#2033,#522,.T.);
#2510=EDGE_CURVE('',#2033,#2033,#1709,.T.);
#2511=EDGE_CURVE('',#2034,#2034,#1710,.T.);
#2512=EDGE_CURVE('',#2034,#2035,#523,.T.);
#2513=EDGE_CURVE('',#2035,#2035,#1711,.T.);
#2514=EDGE_CURVE('',#2036,#2037,#1712,.T.);
#2515=EDGE_CURVE('',#2037,#2036,#1713,.T.);
#2516=EDGE_CURVE('',#2037,#2038,#524,.T.);
#2517=EDGE_CURVE('',#2038,#2038,#1714,.T.);
#2518=EDGE_CURVE('',#2039,#2040,#1715,.T.);
#2519=EDGE_CURVE('',#2040,#2039,#1716,.T.);
#2520=EDGE_CURVE('',#2040,#2041,#525,.T.);
#2521=EDGE_CURVE('',#2041,#2041,#1717,.T.);
#2522=EDGE_CURVE('',#2042,#2042,#1718,.T.);
#2523=EDGE_CURVE('',#2042,#2034,#526,.T.);
#2524=EDGE_CURVE('',#2039,#2043,#527,.T.);
#2525=EDGE_CURVE('',#2043,#2043,#1719,.T.);
#2526=EDGE_CURVE('',#2044,#2044,#1720,.T.);
#2527=EDGE_CURVE('',#2044,#2045,#528,.T.);
#2528=EDGE_CURVE('',#2045,#2045,#1721,.T.);
#2529=EDGE_CURVE('',#2046,#2046,#1722,.T.);
#2530=EDGE_CURVE('',#2046,#2032,#529,.T.);
#2531=EDGE_CURVE('',#2036,#2047,#530,.T.);
#2532=EDGE_CURVE('',#2047,#2047,#1723,.T.);
#2533=EDGE_CURVE('',#2048,#2049,#1724,.T.);
#2534=EDGE_CURVE('',#2050,#2048,#1725,.T.);
#2535=EDGE_CURVE('',#2051,#2050,#1726,.T.);
#2536=EDGE_CURVE('',#2051,#2049,#1727,.T.);
#2537=EDGE_CURVE('',#2052,#2053,#1728,.T.);
#2538=EDGE_CURVE('',#2054,#2052,#1729,.T.);
#2539=EDGE_CURVE('',#2055,#2054,#1730,.T.);
#2540=EDGE_CURVE('',#2055,#2056,#1731,.T.);
#2541=EDGE_CURVE('',#2053,#2056,#1732,.T.);
#2542=EDGE_CURVE('',#2057,#2058,#1733,.T.);
#2543=EDGE_CURVE('',#2059,#2057,#1734,.T.);
#2544=EDGE_CURVE('',#2060,#2059,#1735,.T.);
#2545=EDGE_CURVE('',#2058,#2060,#1736,.T.);
#2546=EDGE_CURVE('',#2061,#2061,#1737,.T.);
#2547=EDGE_CURVE('',#2061,#2062,#531,.T.);
#2548=EDGE_CURVE('',#2062,#2062,#1738,.T.);
#2549=EDGE_CURVE('',#2049,#2063,#532,.T.);
#2550=EDGE_CURVE('',#2064,#2063,#1739,.T.);
#2551=EDGE_CURVE('',#2048,#2064,#533,.T.);
#2552=EDGE_CURVE('',#2065,#2065,#1740,.T.);
#2553=EDGE_CURVE('',#2065,#2066,#534,.T.);
#2554=EDGE_CURVE('',#2066,#2066,#1741,.T.);
#2555=EDGE_CURVE('',#2067,#2068,#1742,.T.);
#2556=EDGE_CURVE('',#2068,#2069,#535,.T.);
#2557=EDGE_CURVE('',#2069,#2070,#1743,.T.);
#2558=EDGE_CURVE('',#2067,#2070,#536,.T.);
#2559=EDGE_CURVE('',#2071,#2071,#1744,.T.);
#2560=EDGE_CURVE('',#2071,#2072,#537,.T.);
#2561=EDGE_CURVE('',#2072,#2073,#1745,.T.);
#2562=EDGE_CURVE('',#2073,#2074,#15,.T.);
#2563=EDGE_CURVE('',#2074,#2075,#16,.T.);
#2564=EDGE_CURVE('',#2076,#2075,#538,.T.);
#2565=EDGE_CURVE('',#2076,#2077,#17,.T.);
#2566=EDGE_CURVE('',#2077,#2052,#18,.T.);
#2567=EDGE_CURVE('',#2053,#2078,#539,.T.);
#2568=EDGE_CURVE('',#2078,#2078,#1746,.T.);
#2569=EDGE_CURVE('',#2056,#2079,#19,.T.);
#2570=EDGE_CURVE('',#2079,#2080,#540,.T.);
#2571=EDGE_CURVE('',#2080,#2081,#20,.T.);
#2572=EDGE_CURVE('',#2081,#2072,#1747,.T.);
#2573=EDGE_CURVE('',#2054,#2082,#541,.T.);
#2574=EDGE_CURVE('',#2082,#2083,#1748,.T.);
#2575=EDGE_CURVE('',#2083,#2084,#542,.T.);
#2576=EDGE_CURVE('',#2084,#2085,#1749,.T.);
#2577=EDGE_CURVE('',#2085,#2086,#543,.T.);
#2578=EDGE_CURVE('',#2086,#2087,#544,.T.);
#2579=EDGE_CURVE('',#2087,#2055,#545,.T.);
#2580=EDGE_CURVE('',#2068,#2076,#546,.T.);
#2581=EDGE_CURVE('',#2075,#2048,#547,.T.);
#2582=EDGE_CURVE('',#2088,#2064,#548,.T.);
#2583=EDGE_CURVE('',#2089,#2088,#549,.T.);
#2584=EDGE_CURVE('',#2089,#2069,#550,.T.);
#2585=EDGE_CURVE('',#2090,#2091,#551,.T.);
#2586=EDGE_CURVE('',#2090,#2067,#552,.T.);
#2587=EDGE_CURVE('',#2070,#2092,#553,.T.);
#2588=EDGE_CURVE('',#2092,#2093,#554,.T.);
#2589=EDGE_CURVE('',#2063,#2093,#555,.T.);
#2590=EDGE_CURVE('',#2049,#2091,#556,.T.);
#2591=EDGE_CURVE('',#2094,#2095,#557,.T.);
#2592=EDGE_CURVE('',#2094,#2090,#1750,.T.);
#2593=EDGE_CURVE('',#2091,#2095,#1751,.T.);
#2594=EDGE_CURVE('',#2058,#2096,#558,.T.);
#2595=EDGE_CURVE('',#2058,#2097,#559,.T.);
#2596=EDGE_CURVE('',#2097,#2098,#1752,.T.);
#2597=EDGE_CURVE('',#2098,#2099,#560,.T.);
#2598=EDGE_CURVE('',#2100,#2099,#1753,.T.);
#2599=EDGE_CURVE('',#2100,#2094,#561,.T.);
#2600=EDGE_CURVE('',#2095,#2101,#562,.T.);
#2601=EDGE_CURVE('',#2102,#2101,#1754,.T.);
#2602=EDGE_CURVE('',#2102,#2103,#563,.T.);
#2603=EDGE_CURVE('',#2103,#2104,#1755,.T.);
#2604=EDGE_CURVE('',#2104,#2105,#564,.T.);
#2605=EDGE_CURVE('',#2105,#2106,#565,.T.);
#2606=EDGE_CURVE('',#2107,#2106,#566,.T.);
#2607=EDGE_CURVE('',#2108,#2107,#567,.T.);
#2608=EDGE_CURVE('',#2108,#2096,#568,.T.);
#2609=EDGE_CURVE('',#2109,#2110,#1756,.T.);
#2610=EDGE_CURVE('',#2110,#2057,#569,.T.);
#2611=EDGE_CURVE('',#2057,#2111,#570,.T.);
#2612=EDGE_CURVE('',#2111,#2112,#571,.T.);
#2613=EDGE_CURVE('',#2112,#2113,#572,.T.);
#2614=EDGE_CURVE('',#2114,#2113,#573,.T.);
#2615=EDGE_CURVE('',#2115,#2114,#574,.T.);
#2616=EDGE_CURVE('',#2115,#2116,#575,.T.);
#2617=EDGE_CURVE('',#2116,#2117,#1757,.T.);
#2618=EDGE_CURVE('',#2117,#2118,#576,.T.);
#2619=EDGE_CURVE('',#2119,#2118,#1758,.T.);
#2620=EDGE_CURVE('',#2119,#2080,#577,.T.);
#2621=EDGE_CURVE('',#2079,#2120,#578,.T.);
#2622=EDGE_CURVE('',#2121,#2120,#1759,.T.);
#2623=EDGE_CURVE('',#2121,#2109,#579,.T.);
#2624=EDGE_CURVE('',#2122,#2123,#580,.T.);
#2625=EDGE_CURVE('',#2123,#2060,#581,.T.);
#2626=EDGE_CURVE('',#2059,#2122,#582,.T.);
#2627=EDGE_CURVE('',#2096,#2111,#1760,.T.);
#2628=EDGE_CURVE('',#2113,#2107,#583,.T.);
#2629=EDGE_CURVE('',#2112,#2108,#584,.T.);
#2630=EDGE_CURVE('',#2093,#2088,#585,.T.);
#2631=EDGE_CURVE('',#2092,#2089,#586,.T.);
#2632=EDGE_CURVE('',#2124,#2125,#587,.T.);
#2633=EDGE_CURVE('',#2125,#2126,#588,.T.);
#2634=EDGE_CURVE('',#2126,#2127,#589,.T.);
#2635=EDGE_CURVE('',#2127,#2124,#590,.T.);
#2636=EDGE_CURVE('',#2128,#2051,#591,.T.);
#2637=EDGE_CURVE('',#2050,#2129,#592,.T.);
#2638=EDGE_CURVE('',#2129,#2130,#1761,.T.);
#2639=EDGE_CURVE('',#2130,#2131,#593,.T.);
#2640=EDGE_CURVE('',#2131,#2132,#594,.T.);
#2641=EDGE_CURVE('',#2132,#2133,#595,.T.);
#2642=EDGE_CURVE('',#2133,#2128,#1762,.T.);
#2643=EDGE_CURVE('',#2134,#2135,#1763,.T.);
#2644=EDGE_CURVE('',#2135,#2136,#596,.T.);
#2645=EDGE_CURVE('',#2136,#2137,#597,.T.);
#2646=EDGE_CURVE('',#2137,#2134,#598,.T.);
#2647=EDGE_CURVE('',#2105,#2115,#1764,.T.);
#2648=EDGE_CURVE('',#2106,#2114,#1765,.T.);
#2649=EDGE_CURVE('',#2138,#2139,#599,.T.);
#2650=EDGE_CURVE('',#2139,#2140,#600,.T.);
#2651=EDGE_CURVE('',#2140,#2141,#601,.T.);
#2652=EDGE_CURVE('',#2141,#2138,#602,.T.);
#2653=EDGE_CURVE('',#2136,#2139,#1766,.T.);
#2654=EDGE_CURVE('',#2138,#2137,#1767,.T.);
#2655=EDGE_CURVE('',#2122,#2125,#1768,.T.);
#2656=EDGE_CURVE('',#2124,#2123,#1769,.T.);
#2657=EDGE_CURVE('',#2122,#2110,#1770,.T.);
#2658=EDGE_CURVE('',#2097,#2123,#1771,.T.);
#2659=EDGE_CURVE('',#2125,#2109,#1772,.T.);
#2660=EDGE_CURVE('',#2098,#2124,#1773,.T.);
#2661=EDGE_CURVE('',#2126,#2121,#1774,.T.);
#2662=EDGE_CURVE('',#2127,#2086,#1775,.T.);
#2663=EDGE_CURVE('',#2087,#2126,#1776,.T.);
#2664=EDGE_CURVE('',#2099,#2127,#1777,.T.);
#2665=EDGE_CURVE('',#2087,#2120,#1778,.T.);
#2666=EDGE_CURVE('',#2100,#2086,#1779,.T.);
#2667=EDGE_CURVE('',#2055,#2079,#21,.T.);
#2668=EDGE_CURVE('',#2094,#2085,#1780,.T.);
#2669=EDGE_CURVE('',#2090,#2084,#1781,.T.);
#2670=EDGE_CURVE('',#2067,#2083,#1782,.T.);
#2671=EDGE_CURVE('',#2054,#2076,#22,.T.);
#2672=EDGE_CURVE('',#2068,#2082,#1783,.T.);
#2673=EDGE_CURVE('',#2135,#2105,#1784,.T.);
#2674=EDGE_CURVE('',#2115,#2134,#1785,.T.);
#2675=EDGE_CURVE('',#2116,#2137,#1786,.T.);
#2676=EDGE_CURVE('',#2136,#2104,#1787,.T.);
#2677=EDGE_CURVE('',#2117,#2138,#1788,.T.);
#2678=EDGE_CURVE('',#2139,#2103,#1789,.T.);
#2679=EDGE_CURVE('',#2118,#2141,#1790,.T.);
#2680=EDGE_CURVE('',#2140,#2102,#1791,.T.);
#2681=EDGE_CURVE('',#2141,#2131,#1792,.T.);
#2682=EDGE_CURVE('',#2132,#2140,#1793,.T.);
#2683=EDGE_CURVE('',#2119,#2131,#1794,.T.);
#2684=EDGE_CURVE('',#2132,#2101,#1795,.T.);
#2685=EDGE_CURVE('',#2080,#2130,#23,.T.);
#2686=EDGE_CURVE('',#2133,#2095,#1796,.T.);
#2687=EDGE_CURVE('',#2081,#2130,#1797,.T.);
#2688=EDGE_CURVE('',#2128,#2091,#1798,.T.);
#2689=EDGE_CURVE('',#2073,#2129,#1799,.T.);
#2690=EDGE_CURVE('',#2075,#2129,#24,.T.);
#3402=ORIENTED_EDGE('',*,*,#2508,.F.);
#3403=ORIENTED_EDGE('',*,*,#2509,.T.);
#3404=ORIENTED_EDGE('',*,*,#2510,.F.);
#3405=ORIENTED_EDGE('',*,*,#2509,.F.);
#3406=ORIENTED_EDGE('',*,*,#2511,.F.);
#3407=ORIENTED_EDGE('',*,*,#2512,.T.);
#3408=ORIENTED_EDGE('',*,*,#2513,.F.);
#3409=ORIENTED_EDGE('',*,*,#2512,.F.);
#3410=ORIENTED_EDGE('',*,*,#2514,.F.);
#3411=ORIENTED_EDGE('',*,*,#2515,.F.);
#3412=ORIENTED_EDGE('',*,*,#2516,.T.);
#3413=ORIENTED_EDGE('',*,*,#2517,.F.);
#3414=ORIENTED_EDGE('',*,*,#2516,.F.);
#3415=ORIENTED_EDGE('',*,*,#2518,.F.);
#3416=ORIENTED_EDGE('',*,*,#2519,.F.);
#3417=ORIENTED_EDGE('',*,*,#2520,.T.);
#3418=ORIENTED_EDGE('',*,*,#2521,.F.);
#3419=ORIENTED_EDGE('',*,*,#2520,.F.);
#3420=ORIENTED_EDGE('',*,*,#2522,.T.);
#3421=ORIENTED_EDGE('',*,*,#2523,.T.);
#3422=ORIENTED_EDGE('',*,*,#2511,.T.);
#3423=ORIENTED_EDGE('',*,*,#2523,.F.);
#3424=ORIENTED_EDGE('',*,*,#2518,.T.);
#3425=ORIENTED_EDGE('',*,*,#2519,.T.);
#3426=ORIENTED_EDGE('',*,*,#2524,.T.);
#3427=ORIENTED_EDGE('',*,*,#2525,.F.);
#3428=ORIENTED_EDGE('',*,*,#2524,.F.);
#3429=ORIENTED_EDGE('',*,*,#2526,.T.);
#3430=ORIENTED_EDGE('',*,*,#2527,.T.);
#3431=ORIENTED_EDGE('',*,*,#2528,.T.);
#3432=ORIENTED_EDGE('',*,*,#2527,.F.);
#3433=ORIENTED_EDGE('',*,*,#2529,.T.);
#3434=ORIENTED_EDGE('',*,*,#2530,.T.);
#3435=ORIENTED_EDGE('',*,*,#2508,.T.);
#3436=ORIENTED_EDGE('',*,*,#2530,.F.);
#3437=ORIENTED_EDGE('',*,*,#2514,.T.);
#3438=ORIENTED_EDGE('',*,*,#2515,.T.);
#3439=ORIENTED_EDGE('',*,*,#2531,.T.);
#3440=ORIENTED_EDGE('',*,*,#2532,.F.);
#3441=ORIENTED_EDGE('',*,*,#2531,.F.);
#3442=ORIENTED_EDGE('',*,*,#2533,.F.);
#3443=ORIENTED_EDGE('',*,*,#2534,.F.);
#3444=ORIENTED_EDGE('',*,*,#2535,.F.);
#3445=ORIENTED_EDGE('',*,*,#2536,.T.);
#3446=ORIENTED_EDGE('',*,*,#2537,.F.);
#3447=ORIENTED_EDGE('',*,*,#2538,.F.);
#3448=ORIENTED_EDGE('',*,*,#2539,.F.);
#3449=ORIENTED_EDGE('',*,*,#2540,.T.);
#3450=ORIENTED_EDGE('',*,*,#2541,.F.);
#3451=ORIENTED_EDGE('',*,*,#2542,.F.);
#3452=ORIENTED_EDGE('',*,*,#2543,.F.);
#3453=ORIENTED_EDGE('',*,*,#2544,.F.);
#3454=ORIENTED_EDGE('',*,*,#2545,.F.);
#3455=ORIENTED_EDGE('',*,*,#2546,.F.);
#3456=ORIENTED_EDGE('',*,*,#2547,.T.);
#3457=ORIENTED_EDGE('',*,*,#2548,.T.);
#3458=ORIENTED_EDGE('',*,*,#2547,.F.);
#3459=ORIENTED_EDGE('',*,*,#2533,.T.);
#3460=ORIENTED_EDGE('',*,*,#2549,.T.);
#3461=ORIENTED_EDGE('',*,*,#2550,.F.);
#3462=ORIENTED_EDGE('',*,*,#2551,.F.);
#3463=ORIENTED_EDGE('',*,*,#2552,.T.);
#3464=ORIENTED_EDGE('',*,*,#2553,.T.);
#3465=ORIENTED_EDGE('',*,*,#2554,.F.);
#3466=ORIENTED_EDGE('',*,*,#2553,.F.);
#3467=ORIENTED_EDGE('',*,*,#2555,.T.);
#3468=ORIENTED_EDGE('',*,*,#2556,.T.);
#3469=ORIENTED_EDGE('',*,*,#2557,.T.);
#3470=ORIENTED_EDGE('',*,*,#2558,.F.);
#3471=ORIENTED_EDGE('',*,*,#2559,.T.);
#3472=ORIENTED_EDGE('',*,*,#2560,.T.);
#3473=ORIENTED_EDGE('',*,*,#2561,.T.);
#3474=ORIENTED_EDGE('',*,*,#2562,.T.);
#3475=ORIENTED_EDGE('',*,*,#2563,.T.);
#3476=ORIENTED_EDGE('',*,*,#2564,.F.);
#3477=ORIENTED_EDGE('',*,*,#2565,.T.);
#3478=ORIENTED_EDGE('',*,*,#2566,.T.);
#3479=ORIENTED_EDGE('',*,*,#2537,.T.);
#3480=ORIENTED_EDGE('',*,*,#2567,.T.);
#3481=ORIENTED_EDGE('',*,*,#2568,.F.);
#3482=ORIENTED_EDGE('',*,*,#2567,.F.);
#3483=ORIENTED_EDGE('',*,*,#2541,.T.);
#3484=ORIENTED_EDGE('',*,*,#2569,.T.);
#3485=ORIENTED_EDGE('',*,*,#2570,.T.);
#3486=ORIENTED_EDGE('',*,*,#2571,.T.);
#3487=ORIENTED_EDGE('',*,*,#2572,.T.);
#3488=ORIENTED_EDGE('',*,*,#2560,.F.);
#3489=ORIENTED_EDGE('',*,*,#2573,.T.);
#3490=ORIENTED_EDGE('',*,*,#2574,.T.);
#3491=ORIENTED_EDGE('',*,*,#2575,.T.);
#3492=ORIENTED_EDGE('',*,*,#2576,.T.);
#3493=ORIENTED_EDGE('',*,*,#2577,.T.);
#3494=ORIENTED_EDGE('',*,*,#2578,.T.);
#3495=ORIENTED_EDGE('',*,*,#2579,.T.);
#3496=ORIENTED_EDGE('',*,*,#2539,.T.);
#3497=ORIENTED_EDGE('',*,*,#2522,.F.);
#3498=ORIENTED_EDGE('',*,*,#2556,.F.);
#3499=ORIENTED_EDGE('',*,*,#2580,.T.);
#3500=ORIENTED_EDGE('',*,*,#2564,.T.);
#3501=ORIENTED_EDGE('',*,*,#2581,.T.);
#3502=ORIENTED_EDGE('',*,*,#2551,.T.);
#3503=ORIENTED_EDGE('',*,*,#2582,.F.);
#3504=ORIENTED_EDGE('',*,*,#2583,.F.);
#3505=ORIENTED_EDGE('',*,*,#2584,.T.);
#3506=ORIENTED_EDGE('',*,*,#2585,.F.);
#3507=ORIENTED_EDGE('',*,*,#2586,.T.);
#3508=ORIENTED_EDGE('',*,*,#2558,.T.);
#3509=ORIENTED_EDGE('',*,*,#2587,.T.);
#3510=ORIENTED_EDGE('',*,*,#2588,.T.);
#3511=ORIENTED_EDGE('',*,*,#2589,.F.);
#3512=ORIENTED_EDGE('',*,*,#2549,.F.);
#3513=ORIENTED_EDGE('',*,*,#2590,.T.);
#3514=ORIENTED_EDGE('',*,*,#2591,.F.);
#3515=ORIENTED_EDGE('',*,*,#2592,.T.);
#3516=ORIENTED_EDGE('',*,*,#2585,.T.);
#3517=ORIENTED_EDGE('',*,*,#2593,.T.);
#3518=ORIENTED_EDGE('',*,*,#2594,.F.);
#3519=ORIENTED_EDGE('',*,*,#2595,.T.);
#3520=ORIENTED_EDGE('',*,*,#2596,.T.);
#3521=ORIENTED_EDGE('',*,*,#2597,.T.);
#3522=ORIENTED_EDGE('',*,*,#2598,.F.);
#3523=ORIENTED_EDGE('',*,*,#2599,.T.);
#3524=ORIENTED_EDGE('',*,*,#2591,.T.);
#3525=ORIENTED_EDGE('',*,*,#2600,.T.);
#3526=ORIENTED_EDGE('',*,*,#2601,.F.);
#3527=ORIENTED_EDGE('',*,*,#2602,.T.);
#3528=ORIENTED_EDGE('',*,*,#2603,.T.);
#3529=ORIENTED_EDGE('',*,*,#2604,.T.);
#3530=ORIENTED_EDGE('',*,*,#2605,.T.);
#3531=ORIENTED_EDGE('',*,*,#2606,.F.);
#3532=ORIENTED_EDGE('',*,*,#2607,.F.);
#3533=ORIENTED_EDGE('',*,*,#2608,.T.);
#3534=ORIENTED_EDGE('',*,*,#2609,.T.);
#3535=ORIENTED_EDGE('',*,*,#2610,.T.);
#3536=ORIENTED_EDGE('',*,*,#2611,.T.);
#3537=ORIENTED_EDGE('',*,*,#2612,.T.);
#3538=ORIENTED_EDGE('',*,*,#2613,.T.);
#3539=ORIENTED_EDGE('',*,*,#2614,.F.);
#3540=ORIENTED_EDGE('',*,*,#2615,.F.);
#3541=ORIENTED_EDGE('',*,*,#2616,.T.);
#3542=ORIENTED_EDGE('',*,*,#2617,.T.);
#3543=ORIENTED_EDGE('',*,*,#2618,.T.);
#3544=ORIENTED_EDGE('',*,*,#2619,.F.);
#3545=ORIENTED_EDGE('',*,*,#2620,.T.);
#3546=ORIENTED_EDGE('',*,*,#2570,.F.);
#3547=ORIENTED_EDGE('',*,*,#2621,.T.);
#3548=ORIENTED_EDGE('',*,*,#2622,.F.);
#3549=ORIENTED_EDGE('',*,*,#2623,.T.);
#3550=ORIENTED_EDGE('',*,*,#2624,.T.);
#3551=ORIENTED_EDGE('',*,*,#2625,.T.);
#3552=ORIENTED_EDGE('',*,*,#2544,.T.);
#3553=ORIENTED_EDGE('',*,*,#2626,.T.);
#3554=ORIENTED_EDGE('',*,*,#2552,.F.);
#3555=ORIENTED_EDGE('',*,*,#2611,.F.);
#3556=ORIENTED_EDGE('',*,*,#2542,.T.);
#3557=ORIENTED_EDGE('',*,*,#2594,.T.);
#3558=ORIENTED_EDGE('',*,*,#2627,.T.);
#3559=ORIENTED_EDGE('',*,*,#2607,.T.);
#3560=ORIENTED_EDGE('',*,*,#2628,.F.);
#3561=ORIENTED_EDGE('',*,*,#2613,.F.);
#3562=ORIENTED_EDGE('',*,*,#2629,.T.);
#3563=ORIENTED_EDGE('',*,*,#2627,.F.);
#3564=ORIENTED_EDGE('',*,*,#2608,.F.);
#3565=ORIENTED_EDGE('',*,*,#2629,.F.);
#3566=ORIENTED_EDGE('',*,*,#2612,.F.);
#3567=ORIENTED_EDGE('',*,*,#2554,.T.);
#3568=ORIENTED_EDGE('',*,*,#2583,.T.);
#3569=ORIENTED_EDGE('',*,*,#2630,.F.);
#3570=ORIENTED_EDGE('',*,*,#2588,.F.);
#3571=ORIENTED_EDGE('',*,*,#2631,.T.);
#3572=ORIENTED_EDGE('',*,*,#2557,.F.);
#3573=ORIENTED_EDGE('',*,*,#2584,.F.);
#3574=ORIENTED_EDGE('',*,*,#2631,.F.);
#3575=ORIENTED_EDGE('',*,*,#2587,.F.);
#3576=ORIENTED_EDGE('',*,*,#2528,.F.);
#3577=ORIENTED_EDGE('',*,*,#2632,.T.);
#3578=ORIENTED_EDGE('',*,*,#2633,.T.);
#3579=ORIENTED_EDGE('',*,*,#2634,.T.);
#3580=ORIENTED_EDGE('',*,*,#2635,.T.);
#3581=ORIENTED_EDGE('',*,*,#2568,.T.);
#3582=ORIENTED_EDGE('',*,*,#2529,.F.);
#3583=ORIENTED_EDGE('',*,*,#2636,.T.);
#3584=ORIENTED_EDGE('',*,*,#2535,.T.);
#3585=ORIENTED_EDGE('',*,*,#2637,.T.);
#3586=ORIENTED_EDGE('',*,*,#2638,.T.);
#3587=ORIENTED_EDGE('',*,*,#2639,.T.);
#3588=ORIENTED_EDGE('',*,*,#2640,.T.);
#3589=ORIENTED_EDGE('',*,*,#2641,.T.);
#3590=ORIENTED_EDGE('',*,*,#2642,.T.);
#3591=ORIENTED_EDGE('',*,*,#2525,.T.);
#3592=ORIENTED_EDGE('',*,*,#2643,.T.);
#3593=ORIENTED_EDGE('',*,*,#2644,.T.);
#3594=ORIENTED_EDGE('',*,*,#2645,.T.);
#3595=ORIENTED_EDGE('',*,*,#2646,.T.);
#3596=ORIENTED_EDGE('',*,*,#2546,.T.);
#3597=ORIENTED_EDGE('',*,*,#2605,.F.);
#3598=ORIENTED_EDGE('',*,*,#2647,.T.);
#3599=ORIENTED_EDGE('',*,*,#2615,.T.);
#3600=ORIENTED_EDGE('',*,*,#2648,.F.);
#3601=ORIENTED_EDGE('',*,*,#2648,.T.);
#3602=ORIENTED_EDGE('',*,*,#2614,.T.);
#3603=ORIENTED_EDGE('',*,*,#2628,.T.);
#3604=ORIENTED_EDGE('',*,*,#2606,.T.);
#3605=ORIENTED_EDGE('',*,*,#2548,.F.);
#3606=ORIENTED_EDGE('',*,*,#2550,.T.);
#3607=ORIENTED_EDGE('',*,*,#2589,.T.);
#3608=ORIENTED_EDGE('',*,*,#2630,.T.);
#3609=ORIENTED_EDGE('',*,*,#2582,.T.);
#3610=ORIENTED_EDGE('',*,*,#2526,.F.);
#3611=ORIENTED_EDGE('',*,*,#2649,.T.);
#3612=ORIENTED_EDGE('',*,*,#2650,.T.);
#3613=ORIENTED_EDGE('',*,*,#2651,.T.);
#3614=ORIENTED_EDGE('',*,*,#2652,.T.);
#3615=ORIENTED_EDGE('',*,*,#2559,.F.);
#3616=ORIENTED_EDGE('',*,*,#2532,.T.);
#3617=ORIENTED_EDGE('',*,*,#2645,.F.);
#3618=ORIENTED_EDGE('',*,*,#2653,.T.);
#3619=ORIENTED_EDGE('',*,*,#2649,.F.);
#3620=ORIENTED_EDGE('',*,*,#2654,.T.);
#3621=ORIENTED_EDGE('',*,*,#2624,.F.);
#3622=ORIENTED_EDGE('',*,*,#2655,.T.);
#3623=ORIENTED_EDGE('',*,*,#2632,.F.);
#3624=ORIENTED_EDGE('',*,*,#2656,.T.);
#3625=ORIENTED_EDGE('',*,*,#2543,.T.);
#3626=ORIENTED_EDGE('',*,*,#2610,.F.);
#3627=ORIENTED_EDGE('',*,*,#2657,.F.);
#3628=ORIENTED_EDGE('',*,*,#2626,.F.);
#3629=ORIENTED_EDGE('',*,*,#2545,.T.);
#3630=ORIENTED_EDGE('',*,*,#2625,.F.);
#3631=ORIENTED_EDGE('',*,*,#2658,.F.);
#3632=ORIENTED_EDGE('',*,*,#2595,.F.);
#3633=ORIENTED_EDGE('',*,*,#2657,.T.);
#3634=ORIENTED_EDGE('',*,*,#2609,.F.);
#3635=ORIENTED_EDGE('',*,*,#2659,.F.);
#3636=ORIENTED_EDGE('',*,*,#2655,.F.);
#3637=ORIENTED_EDGE('',*,*,#2658,.T.);
#3638=ORIENTED_EDGE('',*,*,#2656,.F.);
#3639=ORIENTED_EDGE('',*,*,#2660,.F.);
#3640=ORIENTED_EDGE('',*,*,#2596,.F.);
#3641=ORIENTED_EDGE('',*,*,#2659,.T.);
#3642=ORIENTED_EDGE('',*,*,#2623,.F.);
#3643=ORIENTED_EDGE('',*,*,#2661,.F.);
#3644=ORIENTED_EDGE('',*,*,#2633,.F.);
#3645=ORIENTED_EDGE('',*,*,#2662,.F.);
#3646=ORIENTED_EDGE('',*,*,#2634,.F.);
#3647=ORIENTED_EDGE('',*,*,#2663,.F.);
#3648=ORIENTED_EDGE('',*,*,#2578,.F.);
#3649=ORIENTED_EDGE('',*,*,#2660,.T.);
#3650=ORIENTED_EDGE('',*,*,#2635,.F.);
#3651=ORIENTED_EDGE('',*,*,#2664,.F.);
#3652=ORIENTED_EDGE('',*,*,#2597,.F.);
#3653=ORIENTED_EDGE('',*,*,#2661,.T.);
#3654=ORIENTED_EDGE('',*,*,#2622,.T.);
#3655=ORIENTED_EDGE('',*,*,#2665,.F.);
#3656=ORIENTED_EDGE('',*,*,#2663,.T.);
#3657=ORIENTED_EDGE('',*,*,#2664,.T.);
#3658=ORIENTED_EDGE('',*,*,#2662,.T.);
#3659=ORIENTED_EDGE('',*,*,#2666,.F.);
#3660=ORIENTED_EDGE('',*,*,#2598,.T.);
#3661=ORIENTED_EDGE('',*,*,#2665,.T.);
#3662=ORIENTED_EDGE('',*,*,#2621,.F.);
#3663=ORIENTED_EDGE('',*,*,#2667,.F.);
#3664=ORIENTED_EDGE('',*,*,#2579,.F.);
#3665=ORIENTED_EDGE('',*,*,#2666,.T.);
#3666=ORIENTED_EDGE('',*,*,#2577,.F.);
#3667=ORIENTED_EDGE('',*,*,#2668,.F.);
#3668=ORIENTED_EDGE('',*,*,#2599,.F.);
#3669=ORIENTED_EDGE('',*,*,#2667,.T.);
#3670=ORIENTED_EDGE('',*,*,#2569,.F.);
#3671=ORIENTED_EDGE('',*,*,#2540,.F.);
#3672=ORIENTED_EDGE('',*,*,#2668,.T.);
#3673=ORIENTED_EDGE('',*,*,#2576,.F.);
#3674=ORIENTED_EDGE('',*,*,#2669,.F.);
#3675=ORIENTED_EDGE('',*,*,#2592,.F.);
#3676=ORIENTED_EDGE('',*,*,#2669,.T.);
#3677=ORIENTED_EDGE('',*,*,#2575,.F.);
#3678=ORIENTED_EDGE('',*,*,#2670,.F.);
#3679=ORIENTED_EDGE('',*,*,#2586,.F.);
#3680=ORIENTED_EDGE('',*,*,#2538,.T.);
#3681=ORIENTED_EDGE('',*,*,#2566,.F.);
#3682=ORIENTED_EDGE('',*,*,#2565,.F.);
#3683=ORIENTED_EDGE('',*,*,#2671,.F.);
#3684=ORIENTED_EDGE('',*,*,#2670,.T.);
#3685=ORIENTED_EDGE('',*,*,#2574,.F.);
#3686=ORIENTED_EDGE('',*,*,#2672,.F.);
#3687=ORIENTED_EDGE('',*,*,#2555,.F.);
#3688=ORIENTED_EDGE('',*,*,#2671,.T.);
#3689=ORIENTED_EDGE('',*,*,#2580,.F.);
#3690=ORIENTED_EDGE('',*,*,#2672,.T.);
#3691=ORIENTED_EDGE('',*,*,#2573,.F.);
#3692=ORIENTED_EDGE('',*,*,#2673,.F.);
#3693=ORIENTED_EDGE('',*,*,#2643,.F.);
#3694=ORIENTED_EDGE('',*,*,#2674,.F.);
#3695=ORIENTED_EDGE('',*,*,#2647,.F.);
#3696=ORIENTED_EDGE('',*,*,#2674,.T.);
#3697=ORIENTED_EDGE('',*,*,#2646,.F.);
#3698=ORIENTED_EDGE('',*,*,#2675,.F.);
#3699=ORIENTED_EDGE('',*,*,#2616,.F.);
#3700=ORIENTED_EDGE('',*,*,#2673,.T.);
#3701=ORIENTED_EDGE('',*,*,#2604,.F.);
#3702=ORIENTED_EDGE('',*,*,#2676,.F.);
#3703=ORIENTED_EDGE('',*,*,#2644,.F.);
#3704=ORIENTED_EDGE('',*,*,#2675,.T.);
#3705=ORIENTED_EDGE('',*,*,#2654,.F.);
#3706=ORIENTED_EDGE('',*,*,#2677,.F.);
#3707=ORIENTED_EDGE('',*,*,#2617,.F.);
#3708=ORIENTED_EDGE('',*,*,#2676,.T.);
#3709=ORIENTED_EDGE('',*,*,#2603,.F.);
#3710=ORIENTED_EDGE('',*,*,#2678,.F.);
#3711=ORIENTED_EDGE('',*,*,#2653,.F.);
#3712=ORIENTED_EDGE('',*,*,#2677,.T.);
#3713=ORIENTED_EDGE('',*,*,#2652,.F.);
#3714=ORIENTED_EDGE('',*,*,#2679,.F.);
#3715=ORIENTED_EDGE('',*,*,#2618,.F.);
#3716=ORIENTED_EDGE('',*,*,#2678,.T.);
#3717=ORIENTED_EDGE('',*,*,#2602,.F.);
#3718=ORIENTED_EDGE('',*,*,#2680,.F.);
#3719=ORIENTED_EDGE('',*,*,#2650,.F.);
#3720=ORIENTED_EDGE('',*,*,#2681,.F.);
#3721=ORIENTED_EDGE('',*,*,#2651,.F.);
#3722=ORIENTED_EDGE('',*,*,#2682,.F.);
#3723=ORIENTED_EDGE('',*,*,#2640,.F.);
#3724=ORIENTED_EDGE('',*,*,#2679,.T.);
#3725=ORIENTED_EDGE('',*,*,#2681,.T.);
#3726=ORIENTED_EDGE('',*,*,#2683,.F.);
#3727=ORIENTED_EDGE('',*,*,#2619,.T.);
#3728=ORIENTED_EDGE('',*,*,#2680,.T.);
#3729=ORIENTED_EDGE('',*,*,#2601,.T.);
#3730=ORIENTED_EDGE('',*,*,#2684,.F.);
#3731=ORIENTED_EDGE('',*,*,#2682,.T.);
#3732=ORIENTED_EDGE('',*,*,#2683,.T.);
#3733=ORIENTED_EDGE('',*,*,#2639,.F.);
#3734=ORIENTED_EDGE('',*,*,#2685,.F.);
#3735=ORIENTED_EDGE('',*,*,#2620,.F.);
#3736=ORIENTED_EDGE('',*,*,#2684,.T.);
#3737=ORIENTED_EDGE('',*,*,#2600,.F.);
#3738=ORIENTED_EDGE('',*,*,#2686,.F.);
#3739=ORIENTED_EDGE('',*,*,#2641,.F.);
#3740=ORIENTED_EDGE('',*,*,#2571,.F.);
#3741=ORIENTED_EDGE('',*,*,#2685,.T.);
#3742=ORIENTED_EDGE('',*,*,#2687,.F.);
#3743=ORIENTED_EDGE('',*,*,#2686,.T.);
#3744=ORIENTED_EDGE('',*,*,#2593,.F.);
#3745=ORIENTED_EDGE('',*,*,#2688,.F.);
#3746=ORIENTED_EDGE('',*,*,#2642,.F.);
#3747=ORIENTED_EDGE('',*,*,#2687,.T.);
#3748=ORIENTED_EDGE('',*,*,#2638,.F.);
#3749=ORIENTED_EDGE('',*,*,#2689,.F.);
#3750=ORIENTED_EDGE('',*,*,#2561,.F.);
#3751=ORIENTED_EDGE('',*,*,#2572,.F.);
#3752=ORIENTED_EDGE('',*,*,#2688,.T.);
#3753=ORIENTED_EDGE('',*,*,#2590,.F.);
#3754=ORIENTED_EDGE('',*,*,#2536,.F.);
#3755=ORIENTED_EDGE('',*,*,#2636,.F.);
#3756=ORIENTED_EDGE('',*,*,#2562,.F.);
#3757=ORIENTED_EDGE('',*,*,#2689,.T.);
#3758=ORIENTED_EDGE('',*,*,#2690,.F.);
#3759=ORIENTED_EDGE('',*,*,#2563,.F.);
#3760=ORIENTED_EDGE('',*,*,#2690,.T.);
#3761=ORIENTED_EDGE('',*,*,#2637,.F.);
#3762=ORIENTED_EDGE('',*,*,#2534,.T.);
#3763=ORIENTED_EDGE('',*,*,#2581,.F.);
#3764=ORIENTED_EDGE('',*,*,#2517,.T.);
#3765=ORIENTED_EDGE('',*,*,#2510,.T.);
#3766=ORIENTED_EDGE('',*,*,#2521,.T.);
#3767=ORIENTED_EDGE('',*,*,#2513,.T.);
#3905=TOROIDAL_SURFACE('',#4504,8.,2.);
#3906=TOROIDAL_SURFACE('',#4509,12.,2.);
#3907=TOROIDAL_SURFACE('',#4515,8.,2.);
#3908=TOROIDAL_SURFACE('',#4585,5.,2.);
#3909=TOROIDAL_SURFACE('',#4587,5.,2.);
#3910=TOROIDAL_SURFACE('',#4596,4.,2.);
#3911=TOROIDAL_SURFACE('',#4598,4.,2.);
#3912=TOROIDAL_SURFACE('',#4603,22.,2.);
#3913=TOROIDAL_SURFACE('',#4607,8.,2.);
#3914=TOROIDAL_SURFACE('',#4610,8.,2.);
#3915=TOROIDAL_SURFACE('',#4617,5.,2.);
#3916=TOROIDAL_SURFACE('',#4619,5.,2.);
#3917=TOROIDAL_SURFACE('',#4628,4.,2.);
#3918=TOROIDAL_SURFACE('',#4630,4.,2.);
#3919=TOROIDAL_SURFACE('',#4636,22.,2.);
#3920=TOROIDAL_SURFACE('',#4638,12.,2.);
#4054=ADVANCED_FACE('',(#1219),#104,.T.);
#4055=ADVANCED_FACE('',(#1220),#105,.T.);
#4056=ADVANCED_FACE('',(#1221),#106,.T.);
#4057=ADVANCED_FACE('',(#1222),#107,.T.);
#4058=ADVANCED_FACE('',(#1223),#1045,.T.);
#4059=ADVANCED_FACE('',(#1224),#1046,.T.);
#4060=ADVANCED_FACE('',(#1225),#1047,.T.);
#4061=ADVANCED_FACE('',(#1226),#1048,.T.);
#4062=ADVANCED_FACE('',(#1227),#1049,.T.);
#4063=ADVANCED_FACE('',(#1228),#3905,.T.);
#4064=ADVANCED_FACE('',(#1229),#3906,.F.);
#4065=ADVANCED_FACE('',(#1230),#3907,.T.);
#4066=ADVANCED_FACE('',(#1231),#1050,.F.);
#4067=ADVANCED_FACE('',(#1232),#1051,.T.);
#4068=ADVANCED_FACE('',(#1233),#1052,.F.);
#4069=ADVANCED_FACE('',(#1234),#1053,.T.);
#4070=ADVANCED_FACE('',(#1235),#1054,.T.);
#4071=ADVANCED_FACE('',(#1236,#141),#248,.T.);
#4072=ADVANCED_FACE('',(#1237),#249,.F.);
#4073=ADVANCED_FACE('',(#1238),#250,.F.);
#4074=ADVANCED_FACE('',(#1239),#1055,.F.);
#4075=ADVANCED_FACE('',(#1240),#251,.F.);
#4076=ADVANCED_FACE('',(#1241),#252,.F.);
#4077=ADVANCED_FACE('',(#1242,#142),#253,.T.);
#4078=ADVANCED_FACE('',(#1243),#1056,.T.);
#4079=ADVANCED_FACE('',(#1244),#254,.T.);
#4080=ADVANCED_FACE('',(#1245,#143),#255,.F.);
#4081=ADVANCED_FACE('',(#1246),#256,.T.);
#4082=ADVANCED_FACE('',(#1247,#144),#257,.F.);
#4083=ADVANCED_FACE('',(#1248),#258,.F.);
#4084=ADVANCED_FACE('',(#1249,#145),#259,.T.);
#4085=ADVANCED_FACE('',(#1250,#146),#260,.T.);
#4086=ADVANCED_FACE('',(#1251,#147),#261,.T.);
#4087=ADVANCED_FACE('',(#1252),#1057,.T.);
#4088=ADVANCED_FACE('',(#1253,#148),#262,.F.);
#4089=ADVANCED_FACE('',(#1254,#149),#263,.F.);
#4090=ADVANCED_FACE('',(#1255),#264,.F.);
#4091=ADVANCED_FACE('',(#1256,#150),#265,.T.);
#4092=ADVANCED_FACE('',(#1257),#1058,.T.);
#4093=ADVANCED_FACE('',(#1258),#1059,.T.);
#4094=ADVANCED_FACE('',(#1259),#1060,.T.);
#4095=ADVANCED_FACE('',(#1260),#1061,.T.);
#4096=ADVANCED_FACE('',(#1261),#3908,.T.);
#4097=ADVANCED_FACE('',(#1262),#3909,.T.);
#4098=ADVANCED_FACE('',(#1263),#1062,.T.);
#4099=ADVANCED_FACE('',(#1264),#1063,.F.);
#4100=ADVANCED_FACE('',(#1265),#1064,.T.);
#4101=ADVANCED_FACE('',(#1266),#3910,.T.);
#4102=ADVANCED_FACE('',(#1267),#3911,.T.);
#4103=ADVANCED_FACE('',(#1268),#1065,.T.);
#4104=ADVANCED_FACE('',(#1269),#1066,.T.);
#4105=ADVANCED_FACE('',(#1270),#11,.F.);
#4106=ADVANCED_FACE('',(#1271),#3912,.T.);
#4107=ADVANCED_FACE('',(#1272),#1067,.T.);
#4108=ADVANCED_FACE('',(#1273),#12,.F.);
#4109=ADVANCED_FACE('',(#1274),#3913,.T.);
#4110=ADVANCED_FACE('',(#1275),#1068,.T.);
#4111=ADVANCED_FACE('',(#1276),#3914,.T.);
#4112=ADVANCED_FACE('',(#1277),#1069,.T.);
#4113=ADVANCED_FACE('',(#1278),#1070,.T.);
#4114=ADVANCED_FACE('',(#1279),#3915,.T.);
#4115=ADVANCED_FACE('',(#1280),#3916,.T.);
#4116=ADVANCED_FACE('',(#1281),#1071,.T.);
#4117=ADVANCED_FACE('',(#1282),#1072,.T.);
#4118=ADVANCED_FACE('',(#1283),#1073,.F.);
#4119=ADVANCED_FACE('',(#1284),#3917,.T.);
#4120=ADVANCED_FACE('',(#1285),#3918,.T.);
#4121=ADVANCED_FACE('',(#1286),#1074,.T.);
#4122=ADVANCED_FACE('',(#1287),#1075,.T.);
#4123=ADVANCED_FACE('',(#1288),#13,.F.);
#4124=ADVANCED_FACE('',(#1289),#3919,.T.);
#4125=ADVANCED_FACE('',(#1290),#3920,.F.);
#4126=ADVANCED_FACE('',(#1291),#1076,.T.);
#4127=ADVANCED_FACE('',(#1292),#14,.F.);
#4128=ADVANCED_FACE('',(#1293),#1077,.T.);
#4129=ADVANCED_FACE('',(#1294),#266,.F.);
#4130=ADVANCED_FACE('',(#1295),#267,.T.);
#4131=ADVANCED_FACE('',(#1296),#268,.F.);
#4132=ADVANCED_FACE('',(#1297),#269,.T.);
#4168=CLOSED_SHELL('',(#4054,#4055,#4056,#4057,#4058,#4059,#4060,#4061,
#4062,#4063,#4064,#4065,#4066,#4067,#4068,#4069,#4070,#4071,#4072,#4073,
#4074,#4075,#4076,#4077,#4078,#4079,#4080,#4081,#4082,#4083,#4084,#4085,
#4086,#4087,#4088,#4089,#4090,#4091,#4092,#4093,#4094,#4095,#4096,#4097,
#4098,#4099,#4100,#4101,#4102,#4103,#4104,#4105,#4106,#4107,#4108,#4109,
#4110,#4111,#4112,#4113,#4114,#4115,#4116,#4117,#4118,#4119,#4120,#4121,
#4122,#4123,#4124,#4125,#4126,#4127,#4128,#4129,#4130,#4131,#4132));
#4478=AXIS2_PLACEMENT_3D('',#6669,#5403,#5404);
#4479=AXIS2_PLACEMENT_3D('',#6670,#5405,#5406);
#4480=AXIS2_PLACEMENT_3D('',#6672,#5407,#5408);
#4481=AXIS2_PLACEMENT_3D('',#6675,#5410,#5411);
#4482=AXIS2_PLACEMENT_3D('',#6676,#5412,#5413);
#4483=AXIS2_PLACEMENT_3D('',#6678,#5414,#5415);
#4484=AXIS2_PLACEMENT_3D('',#6681,#5417,#5418);
#4485=AXIS2_PLACEMENT_3D('',#6682,#5419,#5420);
#4486=AXIS2_PLACEMENT_3D('',#6685,#5421,#5422);
#4487=AXIS2_PLACEMENT_3D('',#6686,#5423,#5424);
#4488=AXIS2_PLACEMENT_3D('',#6689,#5426,#5427);
#4489=AXIS2_PLACEMENT_3D('',#6690,#5428,#5429);
#4490=AXIS2_PLACEMENT_3D('',#6693,#5430,#5431);
#4491=AXIS2_PLACEMENT_3D('',#6694,#5432,#5433);
#4492=AXIS2_PLACEMENT_3D('',#6697,#5435,#5436);
#4493=AXIS2_PLACEMENT_3D('',#6698,#5437,#5438);
#4494=AXIS2_PLACEMENT_3D('',#6700,#5439,#5440);
#4495=AXIS2_PLACEMENT_3D('',#6702,#5442,#5443);
#4496=AXIS2_PLACEMENT_3D('',#6705,#5445,#5446);
#4497=AXIS2_PLACEMENT_3D('',#6706,#5447,#5448);
#4498=AXIS2_PLACEMENT_3D('',#6708,#5449,#5450);
#4499=AXIS2_PLACEMENT_3D('',#6711,#5452,#5453);
#4500=AXIS2_PLACEMENT_3D('',#6712,#5454,#5455);
#4501=AXIS2_PLACEMENT_3D('',#6714,#5456,#5457);
#4502=AXIS2_PLACEMENT_3D('',#6716,#5459,#5460);
#4503=AXIS2_PLACEMENT_3D('',#6719,#5462,#5463);
#4504=AXIS2_PLACEMENT_3D('',#6720,#5464,#5465);
#4505=AXIS2_PLACEMENT_3D('',#6723,#5466,#5467);
#4506=AXIS2_PLACEMENT_3D('',#6725,#5468,#5469);
#4507=AXIS2_PLACEMENT_3D('',#6727,#5470,#5471);
#4508=AXIS2_PLACEMENT_3D('',#6728,#5472,#5473);
#4509=AXIS2_PLACEMENT_3D('',#6729,#5474,#5475);
#4510=AXIS2_PLACEMENT_3D('',#6732,#5476,#5477);
#4511=AXIS2_PLACEMENT_3D('',#6734,#5478,#5479);
#4512=AXIS2_PLACEMENT_3D('',#6736,#5480,#5481);
#4513=AXIS2_PLACEMENT_3D('',#6738,#5482,#5483);
#4514=AXIS2_PLACEMENT_3D('',#6739,#5484,#5485);
#4515=AXIS2_PLACEMENT_3D('',#6740,#5486,#5487);
#4516=AXIS2_PLACEMENT_3D('',#6743,#5488,#5489);
#4517=AXIS2_PLACEMENT_3D('',#6745,#5490,#5491);
#4518=AXIS2_PLACEMENT_3D('',#6747,#5492,#5493);
#4519=AXIS2_PLACEMENT_3D('',#6748,#5494,#5495);
#4520=AXIS2_PLACEMENT_3D('',#6749,#5496,#5497);
#4521=AXIS2_PLACEMENT_3D('',#6751,#5498,#5499);
#4522=AXIS2_PLACEMENT_3D('',#6754,#5501,#5502);
#4523=AXIS2_PLACEMENT_3D('',#6755,#5503,#5504);
#4524=AXIS2_PLACEMENT_3D('',#6759,#5506,#5507);
#4525=AXIS2_PLACEMENT_3D('',#6761,#5509,#5510);
#4526=AXIS2_PLACEMENT_3D('',#6763,#5511,#5512);
#4527=AXIS2_PLACEMENT_3D('',#6766,#5514,#5515);
#4528=AXIS2_PLACEMENT_3D('',#6767,#5516,#5517);
#4529=AXIS2_PLACEMENT_3D('',#6770,#5518,#5519);
#4530=AXIS2_PLACEMENT_3D('',#6774,#5521,#5522);
#4531=AXIS2_PLACEMENT_3D('',#6776,#5524,#5525);
#4532=AXIS2_PLACEMENT_3D('',#6778,#5526,#5527);
#4533=AXIS2_PLACEMENT_3D('',#6782,#5529,#5530);
#4534=AXIS2_PLACEMENT_3D('',#6900,#5533,#5534);
#4535=AXIS2_PLACEMENT_3D('',#7036,#5536,#5537);
#4536=AXIS2_PLACEMENT_3D('',#7037,#5538,#5539);
#4537=AXIS2_PLACEMENT_3D('',#7041,#5541,#5542);
#4538=AXIS2_PLACEMENT_3D('',#7045,#5544,#5545);
#4539=AXIS2_PLACEMENT_3D('',#7051,#5549,#5550);
#4540=AXIS2_PLACEMENT_3D('',#7059,#5556,#5557);
#4541=AXIS2_PLACEMENT_3D('',#7070,#5564,#5565);
#4542=AXIS2_PLACEMENT_3D('',#7074,#5567,#5568);
#4543=AXIS2_PLACEMENT_3D('',#7075,#5569,#5570);
#4544=AXIS2_PLACEMENT_3D('',#7076,#5571,#5572);
#4545=AXIS2_PLACEMENT_3D('',#7082,#5575,#5576);
#4546=AXIS2_PLACEMENT_3D('',#7086,#5578,#5579);
#4547=AXIS2_PLACEMENT_3D('',#7091,#5582,#5583);
#4548=AXIS2_PLACEMENT_3D('',#7095,#5585,#5586);
#4549=AXIS2_PLACEMENT_3D('',#7105,#5592,#5593);
#4550=AXIS2_PLACEMENT_3D('',#7108,#5594,#5595);
#4551=AXIS2_PLACEMENT_3D('',#7123,#5603,#5604);
#4552=AXIS2_PLACEMENT_3D('',#7127,#5606,#5607);
#4553=AXIS2_PLACEMENT_3D('',#7132,#5610,#5611);
#4554=AXIS2_PLACEMENT_3D('',#7134,#5613,#5614);
#4555=AXIS2_PLACEMENT_3D('',#7140,#5618,#5619);
#4556=AXIS2_PLACEMENT_3D('',#7141,#5620,#5621);
#4557=AXIS2_PLACEMENT_3D('',#7142,#5622,#5623);
#4558=AXIS2_PLACEMENT_3D('',#7145,#5626,#5627);
#4559=AXIS2_PLACEMENT_3D('',#7146,#5628,#5629);
#4560=AXIS2_PLACEMENT_3D('',#7149,#5632,#5633);
#4561=AXIS2_PLACEMENT_3D('',#7150,#5634,#5635);
#4562=AXIS2_PLACEMENT_3D('',#7159,#5640,#5641);
#4563=AXIS2_PLACEMENT_3D('',#7160,#5642,#5643);
#4564=AXIS2_PLACEMENT_3D('',#7166,#5646,#5647);
#4565=AXIS2_PLACEMENT_3D('',#7173,#5651,#5652);
#4566=AXIS2_PLACEMENT_3D('',#7174,#5653,#5654);
#4567=AXIS2_PLACEMENT_3D('',#7177,#5655,#5656);
#4568=AXIS2_PLACEMENT_3D('',#7183,#5660,#5661);
#4569=AXIS2_PLACEMENT_3D('',#7184,#5662,#5663);
#4570=AXIS2_PLACEMENT_3D('',#7185,#5664,#5665);
#4571=AXIS2_PLACEMENT_3D('',#7186,#5666,#5667);
#4572=AXIS2_PLACEMENT_3D('',#7187,#5668,#5669);
#4573=AXIS2_PLACEMENT_3D('',#7188,#5670,#5671);
#4574=AXIS2_PLACEMENT_3D('',#7197,#5676,#5677);
#4575=AXIS2_PLACEMENT_3D('',#7198,#5678,#5679);
#4576=AXIS2_PLACEMENT_3D('',#7199,#5680,#5681);
#4577=AXIS2_PLACEMENT_3D('',#7200,#5682,#5683);
#4578=AXIS2_PLACEMENT_3D('',#7201,#5684,#5685);
#4579=AXIS2_PLACEMENT_3D('',#7202,#5686,#5687);
#4580=AXIS2_PLACEMENT_3D('',#7203,#5688,#5689);
#4581=AXIS2_PLACEMENT_3D('',#7204,#5690,#5691);
#4582=AXIS2_PLACEMENT_3D('',#7205,#5692,#5693);
#4583=AXIS2_PLACEMENT_3D('',#7206,#5694,#5695);
#4584=AXIS2_PLACEMENT_3D('',#7207,#5696,#5697);
#4585=AXIS2_PLACEMENT_3D('',#7208,#5698,#5699);
#4586=AXIS2_PLACEMENT_3D('',#7209,#5700,#5701);
#4587=AXIS2_PLACEMENT_3D('',#7210,#5702,#5703);
#4588=AXIS2_PLACEMENT_3D('',#7211,#5704,#5705);
#4589=AXIS2_PLACEMENT_3D('',#7212,#5706,#5707);
#4590=AXIS2_PLACEMENT_3D('',#7213,#5708,#5709);
#4591=AXIS2_PLACEMENT_3D('',#7214,#5710,#5711);
#4592=AXIS2_PLACEMENT_3D('',#7215,#5712,#5713);
#4593=AXIS2_PLACEMENT_3D('',#7216,#5714,#5715);
#4594=AXIS2_PLACEMENT_3D('',#7217,#5716,#5717);
#4595=AXIS2_PLACEMENT_3D('',#7218,#5718,#5719);
#4596=AXIS2_PLACEMENT_3D('',#7219,#5720,#5721);
#4597=AXIS2_PLACEMENT_3D('',#7220,#5722,#5723);
#4598=AXIS2_PLACEMENT_3D('',#7221,#5724,#5725);
#4599=AXIS2_PLACEMENT_3D('',#7222,#5726,#5727);
#4600=AXIS2_PLACEMENT_3D('',#7223,#5728,#5729);
#4601=AXIS2_PLACEMENT_3D('',#7240,#5730,#5731);
#4602=AXIS2_PLACEMENT_3D('',#7241,#5732,#5733);
#4603=AXIS2_PLACEMENT_3D('',#7284,#5734,#5735);
#4604=AXIS2_PLACEMENT_3D('',#7285,#5736,#5737);
#4605=AXIS2_PLACEMENT_3D('',#7286,#5738,#5739);
#4606=AXIS2_PLACEMENT_3D('',#7287,#5740,#5741);
#4607=AXIS2_PLACEMENT_3D('',#7346,#5742,#5743);
#4608=AXIS2_PLACEMENT_3D('',#7347,#5744,#5745);
#4609=AXIS2_PLACEMENT_3D('',#7348,#5746,#5747);
#4610=AXIS2_PLACEMENT_3D('',#7349,#5748,#5749);
#4611=AXIS2_PLACEMENT_3D('',#7350,#5750,#5751);
#4612=AXIS2_PLACEMENT_3D('',#7351,#5752,#5753);
#4613=AXIS2_PLACEMENT_3D('',#7352,#5754,#5755);
#4614=AXIS2_PLACEMENT_3D('',#7353,#5756,#5757);
#4615=AXIS2_PLACEMENT_3D('',#7354,#5758,#5759);
#4616=AXIS2_PLACEMENT_3D('',#7355,#5760,#5761);
#4617=AXIS2_PLACEMENT_3D('',#7356,#5762,#5763);
#4618=AXIS2_PLACEMENT_3D('',#7357,#5764,#5765);
#4619=AXIS2_PLACEMENT_3D('',#7358,#5766,#5767);
#4620=AXIS2_PLACEMENT_3D('',#7359,#5768,#5769);
#4621=AXIS2_PLACEMENT_3D('',#7360,#5770,#5771);
#4622=AXIS2_PLACEMENT_3D('',#7361,#5772,#5773);
#4623=AXIS2_PLACEMENT_3D('',#7362,#5774,#5775);
#4624=AXIS2_PLACEMENT_3D('',#7363,#5776,#5777);
#4625=AXIS2_PLACEMENT_3D('',#7364,#5778,#5779);
#4626=AXIS2_PLACEMENT_3D('',#7365,#5780,#5781);
#4627=AXIS2_PLACEMENT_3D('',#7366,#5782,#5783);
#4628=AXIS2_PLACEMENT_3D('',#7367,#5784,#5785);
#4629=AXIS2_PLACEMENT_3D('',#7368,#5786,#5787);
#4630=AXIS2_PLACEMENT_3D('',#7369,#5788,#5789);
#4631=AXIS2_PLACEMENT_3D('',#7370,#5790,#5791);
#4632=AXIS2_PLACEMENT_3D('',#7371,#5792,#5793);
#4633=AXIS2_PLACEMENT_3D('',#7442,#5794,#5795);
#4634=AXIS2_PLACEMENT_3D('',#7443,#5796,#5797);
#4635=AXIS2_PLACEMENT_3D('',#7486,#5798,#5799);
#4636=AXIS2_PLACEMENT_3D('',#7487,#5800,#5801);
#4637=AXIS2_PLACEMENT_3D('',#7488,#5802,#5803);
#4638=AXIS2_PLACEMENT_3D('',#7489,#5804,#5805);
#4639=AXIS2_PLACEMENT_3D('',#7490,#5806,#5807);
#4640=AXIS2_PLACEMENT_3D('',#7491,#5808,#5809);
#4641=AXIS2_PLACEMENT_3D('',#7604,#5810,#5811);
#4642=AXIS2_PLACEMENT_3D('',#7605,#5812,#5813);
#4643=AXIS2_PLACEMENT_3D('',#7606,#5814,#5815);
#4644=AXIS2_PLACEMENT_3D('',#7607,#5816,#5817);
#4645=AXIS2_PLACEMENT_3D('',#7608,#5818,#5819);
#5403=DIRECTION('axis',(0.,0.,1.));
#5404=DIRECTION('refdir',(1.,0.,0.));
#5405=DIRECTION('center_axis',(0.,0.,-1.));
#5406=DIRECTION('ref_axis',(-1.,0.,0.));
#5407=DIRECTION('center_axis',(0.,0.,-1.));
#5408=DIRECTION('ref_axis',(1.,0.,0.));
#5409=DIRECTION('',(-0.707106781186551,8.65956056235497E-17,0.707106781186544));
#5410=DIRECTION('center_axis',(0.,0.,1.));
#5411=DIRECTION('ref_axis',(1.,0.,0.));
#5412=DIRECTION('center_axis',(0.,0.,-1.));
#5413=DIRECTION('ref_axis',(-1.,0.,0.));
#5414=DIRECTION('center_axis',(0.,0.,-1.));
#5415=DIRECTION('ref_axis',(1.,0.,0.));
#5416=DIRECTION('',(-0.707106781186551,8.65956056235498E-17,0.707106781186544));
#5417=DIRECTION('center_axis',(0.,0.,1.));
#5418=DIRECTION('ref_axis',(1.,0.,0.));
#5419=DIRECTION('center_axis',(0.,0.,1.));
#5420=DIRECTION('ref_axis',(1.,0.,0.));
#5421=DIRECTION('center_axis',(0.,0.,1.));
#5422=DIRECTION('ref_axis',(1.,0.,0.));
#5423=DIRECTION('center_axis',(0.,0.,1.));
#5424=DIRECTION('ref_axis',(1.,0.,0.));
#5425=DIRECTION('',(0.707106781186543,8.65956056235488E-17,-0.707106781186551));
#5426=DIRECTION('center_axis',(0.,0.,-1.));
#5427=DIRECTION('ref_axis',(1.,0.,0.));
#5428=DIRECTION('center_axis',(0.,0.,1.));
#5429=DIRECTION('ref_axis',(1.,0.,0.));
#5430=DIRECTION('center_axis',(0.,0.,1.));
#5431=DIRECTION('ref_axis',(1.,0.,0.));
#5432=DIRECTION('center_axis',(0.,0.,1.));
#5433=DIRECTION('ref_axis',(1.,0.,0.));
#5434=DIRECTION('',(0.707106781186543,8.65956056235488E-17,-0.707106781186551));
#5435=DIRECTION('center_axis',(0.,0.,-1.));
#5436=DIRECTION('ref_axis',(1.,0.,0.));
#5437=DIRECTION('center_axis',(0.,0.,-1.));
#5438=DIRECTION('ref_axis',(-1.,0.,0.));
#5439=DIRECTION('center_axis',(0.,0.,1.));
#5440=DIRECTION('ref_axis',(1.,0.,0.));
#5441=DIRECTION('',(0.,0.,1.));
#5442=DIRECTION('center_axis',(0.,0.,-1.));
#5443=DIRECTION('ref_axis',(-1.,0.,0.));
#5444=DIRECTION('',(0.,0.,1.));
#5445=DIRECTION('center_axis',(0.,0.,1.));
#5446=DIRECTION('ref_axis',(-1.,0.,0.));
#5447=DIRECTION('center_axis',(0.,0.,-1.));
#5448=DIRECTION('ref_axis',(-1.,0.,0.));
#5449=DIRECTION('center_axis',(0.,0.,1.));
#5450=DIRECTION('ref_axis',(1.,0.,0.));
#5451=DIRECTION('',(0.,0.,1.));
#5452=DIRECTION('center_axis',(0.,0.,-1.));
#5453=DIRECTION('ref_axis',(1.,0.,0.));
#5454=DIRECTION('center_axis',(0.,0.,-1.));
#5455=DIRECTION('ref_axis',(-1.,0.,0.));
#5456=DIRECTION('center_axis',(0.,0.,1.));
#5457=DIRECTION('ref_axis',(1.,0.,0.));
#5458=DIRECTION('',(0.,0.,1.));
#5459=DIRECTION('center_axis',(0.,0.,-1.));
#5460=DIRECTION('ref_axis',(-1.,0.,0.));
#5461=DIRECTION('',(0.,0.,1.));
#5462=DIRECTION('center_axis',(0.,0.,1.));
#5463=DIRECTION('ref_axis',(-1.,0.,0.));
#5464=DIRECTION('center_axis',(0.,0.,-1.));
#5465=DIRECTION('ref_axis',(-1.,0.,0.));
#5466=DIRECTION('center_axis',(0.,0.,1.));
#5467=DIRECTION('ref_axis',(-1.,0.,0.));
#5468=DIRECTION('center_axis',(0.258819045102526,0.965925826289067,0.));
#5469=DIRECTION('ref_axis',(-0.965925826289067,0.258819045102526,0.));
#5470=DIRECTION('center_axis',(0.,0.,-1.));
#5471=DIRECTION('ref_axis',(-1.,0.,0.));
#5472=DIRECTION('center_axis',(-0.258819045102523,-0.965925826289068,0.));
#5473=DIRECTION('ref_axis',(0.965925826289068,-0.258819045102523,0.));
#5474=DIRECTION('center_axis',(0.,0.,1.));
#5475=DIRECTION('ref_axis',(1.,0.,0.));
#5476=DIRECTION('center_axis',(0.,0.,1.));
#5477=DIRECTION('ref_axis',(1.,0.,0.));
#5478=DIRECTION('center_axis',(0.547412572866653,-0.836862877099655,0.));
#5479=DIRECTION('ref_axis',(0.836862877099655,0.547412572866653,0.));
#5480=DIRECTION('center_axis',(0.,0.,-1.));
#5481=DIRECTION('ref_axis',(1.,-2.66453525910038E-15,0.));
#5482=DIRECTION('center_axis',(-0.666666666666666,0.74535599249993,0.));
#5483=DIRECTION('ref_axis',(-0.74535599249993,-0.666666666666666,0.));
#5484=DIRECTION('center_axis',(0.,0.,1.));
#5485=DIRECTION('ref_axis',(1.,0.,0.));
#5486=DIRECTION('center_axis',(0.,0.,1.));
#5487=DIRECTION('ref_axis',(1.,0.,0.));
#5488=DIRECTION('center_axis',(0.,0.,-1.));
#5489=DIRECTION('ref_axis',(1.,0.,0.));
#5490=DIRECTION('center_axis',(-1.,0.,0.));
#5491=DIRECTION('ref_axis',(0.,0.,1.));
#5492=DIRECTION('center_axis',(0.,0.,1.));
#5493=DIRECTION('ref_axis',(1.,0.,0.));
#5494=DIRECTION('center_axis',(-1.,0.,0.));
#5495=DIRECTION('ref_axis',(0.,0.,1.));
#5496=DIRECTION('center_axis',(0.,0.,1.));
#5497=DIRECTION('ref_axis',(-1.,0.,0.));
#5498=DIRECTION('center_axis',(0.,0.,1.));
#5499=DIRECTION('ref_axis',(1.,0.,0.));
#5500=DIRECTION('',(0.,0.,1.));
#5501=DIRECTION('center_axis',(0.,0.,1.));
#5502=DIRECTION('ref_axis',(1.,0.,0.));
#5503=DIRECTION('center_axis',(0.,0.,1.));
#5504=DIRECTION('ref_axis',(-1.,0.,0.));
#5505=DIRECTION('',(0.,0.,1.));
#5506=DIRECTION('center_axis',(0.,0.,1.));
#5507=DIRECTION('ref_axis',(1.,0.,0.));
#5508=DIRECTION('',(0.,0.,1.));
#5509=DIRECTION('center_axis',(0.,0.,-1.));
#5510=DIRECTION('ref_axis',(-1.,0.,0.));
#5511=DIRECTION('center_axis',(0.,0.,1.));
#5512=DIRECTION('ref_axis',(1.,0.,0.));
#5513=DIRECTION('',(0.,0.,-1.));
#5514=DIRECTION('center_axis',(0.,0.,1.));
#5515=DIRECTION('ref_axis',(1.,0.,0.));
#5516=DIRECTION('center_axis',(0.,0.,-1.));
#5517=DIRECTION('ref_axis',(-1.,0.,0.));
#5518=DIRECTION('center_axis',(0.,0.,-1.));
#5519=DIRECTION('ref_axis',(1.,0.,0.));
#5520=DIRECTION('',(0.,0.,-1.));
#5521=DIRECTION('center_axis',(0.,0.,1.));
#5522=DIRECTION('ref_axis',(1.,0.,0.));
#5523=DIRECTION('',(0.,0.,-1.));
#5524=DIRECTION('center_axis',(0.,0.,-1.));
#5525=DIRECTION('ref_axis',(-1.,0.,0.));
#5526=DIRECTION('center_axis',(0.,0.,1.));
#5527=DIRECTION('ref_axis',(1.,0.,0.));
#5528=DIRECTION('',(0.,0.,1.));
#5529=DIRECTION('center_axis',(0.,0.,-1.));
#5530=DIRECTION('ref_axis',(-1.,0.,0.));
#5531=DIRECTION('',(0.,0.,-1.));
#5532=DIRECTION('',(0.,0.,1.));
#5533=DIRECTION('center_axis',(0.,0.,1.));
#5534=DIRECTION('ref_axis',(1.,0.,0.));
#5535=DIRECTION('',(0.,0.,-1.));
#5536=DIRECTION('center_axis',(0.,0.,-1.));
#5537=DIRECTION('ref_axis',(-1.,0.,0.));
#5538=DIRECTION('center_axis',(0.,0.,1.));
#5539=DIRECTION('ref_axis',(1.,0.,0.));
#5540=DIRECTION('',(-0.258819045102525,-0.965925826289067,0.));
#5541=DIRECTION('center_axis',(0.,0.,1.));
#5542=DIRECTION('ref_axis',(1.,0.,0.));
#5543=DIRECTION('',(0.258819045102524,0.965925826289067,0.));
#5544=DIRECTION('center_axis',(0.,0.,-1.));
#5545=DIRECTION('ref_axis',(1.,0.,0.));
#5546=DIRECTION('',(1.,-6.088865147686E-17,0.));
#5547=DIRECTION('',(-3.46944695195361E-16,1.,0.));
#5548=DIRECTION('',(-1.,0.,0.));
#5549=DIRECTION('center_axis',(0.965925826289067,-0.258819045102525,0.));
#5550=DIRECTION('ref_axis',(0.258819045102525,0.965925826289067,0.));
#5551=DIRECTION('',(0.258819045102525,0.965925826289067,0.));
#5552=DIRECTION('',(-0.258819045102525,-0.965925826289067,0.));
#5553=DIRECTION('',(-0.258819045102525,-0.965925826289067,0.));
#5554=DIRECTION('',(0.,0.,-1.));
#5555=DIRECTION('',(-0.258819045102525,-0.965925826289067,0.));
#5556=DIRECTION('center_axis',(-0.965925826289067,0.258819045102524,0.));
#5557=DIRECTION('ref_axis',(-0.258819045102524,-0.965925826289067,0.));
#5558=DIRECTION('',(0.,0.,-1.));
#5559=DIRECTION('',(-0.258819045102524,-0.965925826289067,0.));
#5560=DIRECTION('',(0.258819045102524,0.965925826289067,0.));
#5561=DIRECTION('',(0.,0.,-1.));
#5562=DIRECTION('',(0.258819045102524,0.965925826289067,0.));
#5563=DIRECTION('',(0.258819045102524,0.965925826289067,0.));
#5564=DIRECTION('center_axis',(0.,0.,-1.));
#5565=DIRECTION('ref_axis',(-1.,0.,0.));
#5566=DIRECTION('',(0.,0.,-1.));
#5567=DIRECTION('center_axis',(0.,0.,1.));
#5568=DIRECTION('ref_axis',(1.,0.,0.));
#5569=DIRECTION('center_axis',(0.,0.,-1.));
#5570=DIRECTION('ref_axis',(-1.,0.,0.));
#5571=DIRECTION('center_axis',(6.088865147686E-17,1.,0.));
#5572=DIRECTION('ref_axis',(-1.,6.088865147686E-17,0.));
#5573=DIRECTION('',(0.,0.,-1.));
#5574=DIRECTION('',(-1.,6.088865147686E-17,0.));
#5575=DIRECTION('center_axis',(-6.088865147686E-17,-1.,0.));
#5576=DIRECTION('ref_axis',(-1.,6.088865147686E-17,0.));
#5577=DIRECTION('',(0.,0.,-1.));
#5578=DIRECTION('center_axis',(-6.088865147686E-17,-1.,0.));
#5579=DIRECTION('ref_axis',(-1.,6.088865147686E-17,0.));
#5580=DIRECTION('',(-1.,6.088865147686E-17,0.));
#5581=DIRECTION('',(1.,-6.088865147686E-17,0.));
#5582=DIRECTION('center_axis',(-6.088865147686E-17,-1.,0.));
#5583=DIRECTION('ref_axis',(-1.,6.088865147686E-17,0.));
#5584=DIRECTION('',(0.,0.,-1.));
#5585=DIRECTION('center_axis',(-6.088865147686E-17,-1.,0.));
#5586=DIRECTION('ref_axis',(-1.,6.088865147686E-17,0.));
#5587=DIRECTION('',(1.,-6.088865147686E-17,0.));
#5588=DIRECTION('',(0.,0.,1.));
#5589=DIRECTION('',(1.,-6.67201336914156E-17,0.));
#5590=DIRECTION('',(0.,0.,-1.));
#5591=DIRECTION('',(1.,-6.67201336914156E-17,0.));
#5592=DIRECTION('center_axis',(0.,-1.,0.));
#5593=DIRECTION('ref_axis',(0.,0.,-1.));
#5594=DIRECTION('center_axis',(0.,1.,0.));
#5595=DIRECTION('ref_axis',(0.,0.,-1.));
#5596=DIRECTION('',(1.,0.,0.));
#5597=DIRECTION('',(0.,0.,-1.));
#5598=DIRECTION('',(-1.,0.,0.));
#5599=DIRECTION('',(0.,0.,-1.));
#5600=DIRECTION('',(-1.,0.,0.));
#5601=DIRECTION('',(0.,0.,1.));
#5602=DIRECTION('',(-1.,0.,0.));
#5603=DIRECTION('center_axis',(0.,1.,0.));
#5604=DIRECTION('ref_axis',(0.,0.,-1.));
#5605=DIRECTION('',(0.,0.,1.));
#5606=DIRECTION('center_axis',(0.,1.,0.));
#5607=DIRECTION('ref_axis',(0.,0.,-1.));
#5608=DIRECTION('',(-1.,0.,0.));
#5609=DIRECTION('',(1.,0.,0.));
#5610=DIRECTION('center_axis',(0.,1.,0.));
#5611=DIRECTION('ref_axis',(0.,0.,-1.));
#5612=DIRECTION('',(0.,0.,1.));
#5613=DIRECTION('center_axis',(0.,0.,1.));
#5614=DIRECTION('ref_axis',(1.,0.,0.));
#5615=DIRECTION('',(3.46944695195361E-16,-1.,0.));
#5616=DIRECTION('',(1.,-6.088865147686E-17,0.));
#5617=DIRECTION('',(-1.,0.,0.));
#5618=DIRECTION('center_axis',(0.,0.,-1.));
#5619=DIRECTION('ref_axis',(1.,1.22464679914735E-16,0.));
#5620=DIRECTION('center_axis',(0.,0.,1.));
#5621=DIRECTION('ref_axis',(1.,0.,0.));
#5622=DIRECTION('center_axis',(1.,-3.46944695195361E-16,0.));
#5623=DIRECTION('ref_axis',(3.46944695195361E-16,1.,0.));
#5624=DIRECTION('',(-3.46944695195361E-16,-1.,0.));
#5625=DIRECTION('',(-3.46944695195361E-16,-1.,0.));
#5626=DIRECTION('center_axis',(0.,0.,1.));
#5627=DIRECTION('ref_axis',(1.,0.,0.));
#5628=DIRECTION('center_axis',(-0.258819045102524,-0.965925826289067,0.));
#5629=DIRECTION('ref_axis',(0.965925826289067,-0.258819045102524,0.));
#5630=DIRECTION('',(-0.965925826289067,0.258819045102524,0.));
#5631=DIRECTION('',(-0.965925826289067,0.258819045102524,0.));
#5632=DIRECTION('center_axis',(0.,0.,1.));
#5633=DIRECTION('ref_axis',(1.,0.,0.));
#5634=DIRECTION('center_axis',(1.,3.46944695195361E-16,0.));
#5635=DIRECTION('ref_axis',(-3.46944695195361E-16,1.,0.));
#5636=DIRECTION('',(-3.46944695195361E-16,1.,0.));
#5637=DIRECTION('',(0.,0.,-1.));
#5638=DIRECTION('',(3.46944695195361E-16,-1.,0.));
#5639=DIRECTION('',(0.,0.,1.));
#5640=DIRECTION('center_axis',(0.,0.,1.));
#5641=DIRECTION('ref_axis',(1.,0.,0.));
#5642=DIRECTION('center_axis',(0.,0.,-1.));
#5643=DIRECTION('ref_axis',(1.,0.,0.));
#5644=DIRECTION('',(-0.258819045102524,-0.965925826289067,0.));
#5645=DIRECTION('',(0.258819045102525,0.965925826289067,0.));
#5646=DIRECTION('center_axis',(0.,0.,1.));
#5647=DIRECTION('ref_axis',(-1.,0.,0.));
#5648=DIRECTION('',(1.,0.,0.));
#5649=DIRECTION('',(3.46944695195361E-16,-1.,0.));
#5650=DIRECTION('',(-1.,6.088865147686E-17,0.));
#5651=DIRECTION('center_axis',(0.,0.,1.));
#5652=DIRECTION('ref_axis',(-1.,9.46212805078258E-16,0.));
#5653=DIRECTION('center_axis',(0.,0.,-1.));
#5654=DIRECTION('ref_axis',(1.,0.,0.));
#5655=DIRECTION('center_axis',(0.,0.,-1.));
#5656=DIRECTION('ref_axis',(-1.,0.,0.));
#5657=DIRECTION('',(-1.,6.088865147686E-17,0.));
#5658=DIRECTION('',(-3.46944695195361E-16,1.,0.));
#5659=DIRECTION('',(1.,0.,0.));
#5660=DIRECTION('center_axis',(0.,0.,1.));
#5661=DIRECTION('ref_axis',(1.,-1.22464679914735E-16,0.));
#5662=DIRECTION('center_axis',(0.,0.,1.));
#5663=DIRECTION('ref_axis',(-1.,0.,0.));
#5664=DIRECTION('center_axis',(0.,0.,1.));
#5665=DIRECTION('ref_axis',(1.,0.,0.));
#5666=DIRECTION('center_axis',(0.,0.,-1.));
#5667=DIRECTION('ref_axis',(1.,0.,0.));
#5668=DIRECTION('center_axis',(0.,0.,-1.));
#5669=DIRECTION('ref_axis',(1.,0.,0.));
#5670=DIRECTION('center_axis',(1.,3.46944695195361E-16,0.));
#5671=DIRECTION('ref_axis',(-3.46944695195361E-16,1.,0.));
#5672=DIRECTION('',(3.46944695195361E-16,-1.,0.));
#5673=DIRECTION('',(0.,0.,1.));
#5674=DIRECTION('',(-3.46944695195361E-16,1.,0.));
#5675=DIRECTION('',(0.,0.,-1.));
#5676=DIRECTION('center_axis',(0.,0.,-1.));
#5677=DIRECTION('ref_axis',(1.,0.,0.));
#5678=DIRECTION('center_axis',(3.46944695195361E-16,-1.,0.));
#5679=DIRECTION('ref_axis',(1.,3.46944695195361E-16,0.));
#5680=DIRECTION('center_axis',(6.088865147686E-17,1.,0.));
#5681=DIRECTION('ref_axis',(-1.,6.088865147686E-17,0.));
#5682=DIRECTION('center_axis',(0.,-1.,0.));
#5683=DIRECTION('ref_axis',(0.,0.,-1.));
#5684=DIRECTION('center_axis',(3.46944695195361E-16,-1.,0.));
#5685=DIRECTION('ref_axis',(1.,3.46944695195361E-16,0.));
#5686=DIRECTION('center_axis',(0.,-1.,0.));
#5687=DIRECTION('ref_axis',(0.,0.,-1.));
#5688=DIRECTION('center_axis',(6.088865147686E-17,1.,0.));
#5689=DIRECTION('ref_axis',(-1.,6.088865147686E-17,0.));
#5690=DIRECTION('center_axis',(1.,0.,0.));
#5691=DIRECTION('ref_axis',(0.,0.,-1.));
#5692=DIRECTION('center_axis',(-1.,0.,0.));
#5693=DIRECTION('ref_axis',(0.,0.,1.));
#5694=DIRECTION('center_axis',(-1.,6.088865147686E-17,0.));
#5695=DIRECTION('ref_axis',(-6.088865147686E-17,-1.,0.));
#5696=DIRECTION('center_axis',(-1.,0.,0.));
#5697=DIRECTION('ref_axis',(0.,0.,1.));
#5698=DIRECTION('center_axis',(0.,-1.,0.));
#5699=DIRECTION('ref_axis',(0.,0.,-1.));
#5700=DIRECTION('center_axis',(0.,0.,-1.));
#5701=DIRECTION('ref_axis',(-1.,0.,0.));
#5702=DIRECTION('center_axis',(6.088865147686E-17,1.,0.));
#5703=DIRECTION('ref_axis',(-1.,0.,0.));
#5704=DIRECTION('center_axis',(0.,0.,-1.));
#5705=DIRECTION('ref_axis',(-1.,0.,0.));
#5706=DIRECTION('center_axis',(0.,0.,1.));
#5707=DIRECTION('ref_axis',(1.,0.,0.));
#5708=DIRECTION('center_axis',(0.,0.,-1.));
#5709=DIRECTION('ref_axis',(-1.,0.,0.));
#5710=DIRECTION('center_axis',(-3.46944695195361E-16,1.,0.));
#5711=DIRECTION('ref_axis',(-1.,-3.46944695195361E-16,0.));
#5712=DIRECTION('center_axis',(6.088865147686E-17,1.,0.));
#5713=DIRECTION('ref_axis',(-1.,6.088865147686E-17,0.));
#5714=DIRECTION('center_axis',(0.,-1.,0.));
#5715=DIRECTION('ref_axis',(0.,0.,-1.));
#5716=DIRECTION('center_axis',(0.,0.,1.));
#5717=DIRECTION('ref_axis',(1.,0.,0.));
#5718=DIRECTION('center_axis',(0.,0.,-1.));
#5719=DIRECTION('ref_axis',(-1.,0.,0.));
#5720=DIRECTION('center_axis',(0.,-1.,0.));
#5721=DIRECTION('ref_axis',(0.,0.,-1.));
#5722=DIRECTION('center_axis',(-1.,0.,0.));
#5723=DIRECTION('ref_axis',(0.,0.,-1.));
#5724=DIRECTION('center_axis',(6.088865147686E-17,1.,0.));
#5725=DIRECTION('ref_axis',(-1.,0.,0.));
#5726=DIRECTION('center_axis',(-1.,0.,0.));
#5727=DIRECTION('ref_axis',(0.,0.,-1.));
#5728=DIRECTION('center_axis',(1.,0.,0.));
#5729=DIRECTION('ref_axis',(0.,0.,-1.));
#5730=DIRECTION('center_axis',(-1.,6.088865147686E-17,0.));
#5731=DIRECTION('ref_axis',(-6.088865147686E-17,-1.,0.));
#5732=DIRECTION('center_axis',(-1.,0.,0.));
#5733=DIRECTION('ref_axis',(0.,0.,1.));
#5734=DIRECTION('center_axis',(0.,0.,1.));
#5735=DIRECTION('ref_axis',(1.,0.,0.));
#5736=DIRECTION('center_axis',(-0.258819045102525,-0.965925826289067,5.8928555905964E-16));
#5737=DIRECTION('ref_axis',(0.965925826289067,-0.258819045102525,-3.84362793942457E-32));
#5738=DIRECTION('center_axis',(-0.258819045102524,-0.965925826289067,0.));
#5739=DIRECTION('ref_axis',(0.965925826289067,-0.258819045102524,0.));
#5740=DIRECTION('center_axis',(-0.258819045102523,-0.965925826289068,-5.61224341961558E-17));
#5741=DIRECTION('ref_axis',(0.965925826289068,-0.258819045102523,-2.72649669415818E-33));
#5742=DIRECTION('center_axis',(0.,0.,1.));
#5743=DIRECTION('ref_axis',(-0.258819045102525,-0.965925826289067,0.));
#5744=DIRECTION('center_axis',(0.258819045102526,0.965925826289067,4.48979473569252E-16));
#5745=DIRECTION('ref_axis',(-0.965925826289067,0.258819045102526,-1.81510300540188E-31));
#5746=DIRECTION('center_axis',(0.258819045102525,0.965925826289067,0.));
#5747=DIRECTION('ref_axis',(-0.965925826289067,0.258819045102525,0.));
#5748=DIRECTION('center_axis',(0.,0.,-1.));
#5749=DIRECTION('ref_axis',(1.,-1.22464679914735E-16,0.));
#5750=DIRECTION('center_axis',(-1.,0.,0.));
#5751=DIRECTION('ref_axis',(0.,0.,1.));
#5752=DIRECTION('center_axis',(-1.,0.,0.));
#5753=DIRECTION('ref_axis',(0.,0.,1.));
#5754=DIRECTION('center_axis',(1.,0.,0.));
#5755=DIRECTION('ref_axis',(0.,0.,-1.));
#5756=DIRECTION('center_axis',(-1.,0.,0.));
#5757=DIRECTION('ref_axis',(0.,0.,1.));
#5758=DIRECTION('center_axis',(-1.,6.088865147686E-17,0.));
#5759=DIRECTION('ref_axis',(-6.088865147686E-17,-1.,0.));
#5760=DIRECTION('center_axis',(-1.,0.,0.));
#5761=DIRECTION('ref_axis',(0.,0.,1.));
#5762=DIRECTION('center_axis',(0.,-1.,0.));
#5763=DIRECTION('ref_axis',(0.,0.,-1.));
#5764=DIRECTION('center_axis',(0.,0.,1.));
#5765=DIRECTION('ref_axis',(1.,0.,0.));
#5766=DIRECTION('center_axis',(6.088865147686E-17,1.,0.));
#5767=DIRECTION('ref_axis',(-1.,0.,0.));
#5768=DIRECTION('center_axis',(0.,0.,1.));
#5769=DIRECTION('ref_axis',(1.,0.,0.));
#5770=DIRECTION('center_axis',(0.,0.,-1.));
#5771=DIRECTION('ref_axis',(-1.,0.,0.));
#5772=DIRECTION('center_axis',(0.,0.,1.));
#5773=DIRECTION('ref_axis',(1.,0.,0.));
#5774=DIRECTION('center_axis',(0.,0.,-1.));
#5775=DIRECTION('ref_axis',(-1.,0.,0.));
#5776=DIRECTION('center_axis',(0.,0.,1.));
#5777=DIRECTION('ref_axis',(1.,0.,0.));
#5778=DIRECTION('center_axis',(-3.46944695195361E-16,1.,0.));
#5779=DIRECTION('ref_axis',(-1.,-3.46944695195361E-16,0.));
#5780=DIRECTION('center_axis',(0.,-1.,0.));
#5781=DIRECTION('ref_axis',(0.,0.,-1.));
#5782=DIRECTION('center_axis',(6.088865147686E-17,1.,0.));
#5783=DIRECTION('ref_axis',(-1.,6.088865147686E-17,0.));
#5784=DIRECTION('center_axis',(0.,-1.,0.));
#5785=DIRECTION('ref_axis',(0.,0.,-1.));
#5786=DIRECTION('center_axis',(-1.,0.,0.));
#5787=DIRECTION('ref_axis',(0.,0.,-1.));
#5788=DIRECTION('center_axis',(6.088865147686E-17,1.,0.));
#5789=DIRECTION('ref_axis',(-1.,0.,0.));
#5790=DIRECTION('center_axis',(-1.,0.,0.));
#5791=DIRECTION('ref_axis',(0.,0.,-1.));
#5792=DIRECTION('center_axis',(1.,0.,0.));
#5793=DIRECTION('ref_axis',(0.,0.,-1.));
#5794=DIRECTION('center_axis',(-1.,6.088865147686E-17,0.));
#5795=DIRECTION('ref_axis',(-6.088865147686E-17,-1.,0.));
#5796=DIRECTION('center_axis',(-1.,0.,0.));
#5797=DIRECTION('ref_axis',(0.,0.,1.));
#5798=DIRECTION('center_axis',(-0.666666666666667,0.74535599249993,5.78241158658935E-16));
#5799=DIRECTION('ref_axis',(-0.74535599249993,-0.666666666666667,6.22764116085459E-33));
#5800=DIRECTION('center_axis',(0.,0.,-1.));
#5801=DIRECTION('ref_axis',(-1.,0.,0.));
#5802=DIRECTION('center_axis',(-0.258819045102525,-0.965925826289067,0.));
#5803=DIRECTION('ref_axis',(0.965925826289067,-0.258819045102525,0.));
#5804=DIRECTION('center_axis',(0.,0.,-1.));
#5805=DIRECTION('ref_axis',(0.608761429008719,-0.793353340291237,0.));
#5806=DIRECTION('center_axis',(0.547412572866653,-0.836862877099655,-4.74804720598323E-16));
#5807=DIRECTION('ref_axis',(0.836862877099655,0.547412572866653,-7.02765767035438E-33));
#5808=DIRECTION('center_axis',(-0.258819045102524,-0.965925826289067,0.));
#5809=DIRECTION('ref_axis',(0.965925826289067,-0.258819045102524,0.));
#5810=DIRECTION('center_axis',(0.258819045102525,0.965925826289067,0.));
#5811=DIRECTION('ref_axis',(-0.965925826289067,0.258819045102525,0.));
#5812=DIRECTION('center_axis',(0.,0.,1.));
#5813=DIRECTION('ref_axis',(1.,0.,0.));
#5814=DIRECTION('center_axis',(0.,0.,1.));
#5815=DIRECTION('ref_axis',(1.,0.,0.));
#5816=DIRECTION('center_axis',(0.,0.,1.));
#5817=DIRECTION('ref_axis',(1.,0.,0.));
#5818=DIRECTION('center_axis',(0.,0.,1.));
#5819=DIRECTION('ref_axis',(1.,0.,0.));
#6669=CARTESIAN_POINT('',(0.,0.,0.));
#6670=CARTESIAN_POINT('Origin',(0.,0.,25.));
#6671=CARTESIAN_POINT('',(5.,-6.12323399573676E-16,24.));
#6672=CARTESIAN_POINT('Origin',(0.,0.,24.));
#6673=CARTESIAN_POINT('',(3.99999999999998,-4.89858719658939E-16,25.));
#6674=CARTESIAN_POINT('',(3.99999999999998,-4.89858719658939E-16,25.));
#6675=CARTESIAN_POINT('Origin',(0.,0.,25.));
#6676=CARTESIAN_POINT('Origin',(-10.352761804101,-38.6370330515627,13.));
#6677=CARTESIAN_POINT('',(-5.35276180410099,-38.6370330515627,12.));
#6678=CARTESIAN_POINT('Origin',(-10.352761804101,-38.6370330515627,12.));
#6679=CARTESIAN_POINT('',(-6.35276180410101,-38.6370330515627,13.));
#6680=CARTESIAN_POINT('',(-6.35276180410101,-38.6370330515627,13.));
#6681=CARTESIAN_POINT('Origin',(-10.352761804101,-38.6370330515627,13.));
#6682=CARTESIAN_POINT('Origin',(0.,0.,-24.));
#6683=CARTESIAN_POINT('',(5.,6.12323399573676E-16,-24.));
#6684=CARTESIAN_POINT('',(-5.,-6.12323399573676E-16,-24.));
#6685=CARTESIAN_POINT('Origin',(0.,0.,-24.));
#6686=CARTESIAN_POINT('Origin',(0.,0.,-24.));
#6687=CARTESIAN_POINT('',(-3.99999999999999,-4.8985871965894E-16,-25.));
#6688=CARTESIAN_POINT('',(-5.,-6.12323399573676E-16,-24.));
#6689=CARTESIAN_POINT('Origin',(0.,0.,-25.));
#6690=CARTESIAN_POINT('Origin',(-10.352761804101,-38.6370330515627,-12.));
#6691=CARTESIAN_POINT('',(-5.35276180410099,-38.6370330515627,-12.));
#6692=CARTESIAN_POINT('',(-15.352761804101,-38.6370330515627,-12.));
#6693=CARTESIAN_POINT('Origin',(-10.352761804101,-38.6370330515627,-12.));
#6694=CARTESIAN_POINT('Origin',(-10.352761804101,-38.6370330515627,-12.));
#6695=CARTESIAN_POINT('',(-14.352761804101,-38.6370330515627,-13.));
#6696=CARTESIAN_POINT('',(-15.352761804101,-38.6370330515627,-12.));
#6697=CARTESIAN_POINT('Origin',(-10.352761804101,-38.6370330515627,-13.));
#6698=CARTESIAN_POINT('Origin',(-10.352761804101,-38.6370330515627,13.));
#6699=CARTESIAN_POINT('',(-5.35276180410099,-38.6370330515627,10.));
#6700=CARTESIAN_POINT('Origin',(-10.352761804101,-38.6370330515627,10.));
#6701=CARTESIAN_POINT('',(-5.35276180410099,-38.6370330515627,13.));
#6702=CARTESIAN_POINT('Origin',(-10.352761804101,-38.6370330515627,13.));
#6703=CARTESIAN_POINT('',(-5.35276180410099,-38.6370330515627,-10.));
#6704=CARTESIAN_POINT('',(-5.35276180410099,-38.6370330515627,13.));
#6705=CARTESIAN_POINT('Origin',(-10.352761804101,-38.6370330515627,-10.));
#6706=CARTESIAN_POINT('Origin',(-10.352761804101,-38.6370330515627,13.));
#6707=CARTESIAN_POINT('',(-5.35276180410099,-38.6370330515627,-5.));
#6708=CARTESIAN_POINT('Origin',(-10.352761804101,-38.6370330515627,-5.));
#6709=CARTESIAN_POINT('',(-5.35276180410099,-38.6370330515627,5.));
#6710=CARTESIAN_POINT('',(-5.35276180410099,-38.6370330515627,13.));
#6711=CARTESIAN_POINT('Origin',(-10.352761804101,-38.6370330515627,5.));
#6712=CARTESIAN_POINT('Origin',(0.,0.,25.));
#6713=CARTESIAN_POINT('',(5.,-6.12323399573676E-16,15.));
#6714=CARTESIAN_POINT('Origin',(0.,0.,15.));
#6715=CARTESIAN_POINT('',(5.,-6.12323399573676E-16,25.));
#6716=CARTESIAN_POINT('Origin',(0.,0.,25.));
#6717=CARTESIAN_POINT('',(5.,-6.12323399573676E-16,-15.));
#6718=CARTESIAN_POINT('',(5.,-6.12323399573676E-16,25.));
#6719=CARTESIAN_POINT('Origin',(0.,0.,-15.));
#6720=CARTESIAN_POINT('Origin',(-10.352761804101,-38.6370330515627,-8.));
#6721=CARTESIAN_POINT('',(-20.0120200669917,-36.0488426005374,-8.));
#6722=CARTESIAN_POINT('',(-0.693503541210314,-41.2252235025879,-8.));
#6723=CARTESIAN_POINT('Origin',(-10.352761804101,-38.6370330515627,-8.));
#6724=CARTESIAN_POINT('',(-18.0801684144135,-36.5664806907425,-10.));
#6725=CARTESIAN_POINT('Origin',(-18.0801684144135,-36.5664806907425,-8.));
#6726=CARTESIAN_POINT('',(-2.62535519378845,-40.7075854123829,-10.));
#6727=CARTESIAN_POINT('Origin',(-10.352761804101,-38.6370330515627,-10.));
#6728=CARTESIAN_POINT('Origin',(-2.62535519378845,-40.7075854123829,-8.));
#6729=CARTESIAN_POINT('Origin',(0.,0.,12.));
#6730=CARTESIAN_POINT('',(-8.36862877099655,-5.47412572866653,12.));
#6731=CARTESIAN_POINT('',(10.,-1.22464679914735E-15,12.));
#6732=CARTESIAN_POINT('Origin',(0.,0.,12.));
#6733=CARTESIAN_POINT('',(-10.0423545251959,-6.56895087439983,10.));
#6734=CARTESIAN_POINT('Origin',(-10.0423545251959,-6.56895087439983,12.));
#6735=CARTESIAN_POINT('',(8.94427190999916,8.,10.));
#6736=CARTESIAN_POINT('Origin',(0.,0.,10.));
#6737=CARTESIAN_POINT('',(7.4535599249993,6.66666666666667,12.));
#6738=CARTESIAN_POINT('Origin',(8.94427190999916,8.,12.));
#6739=CARTESIAN_POINT('Origin',(0.,0.,12.));
#6740=CARTESIAN_POINT('Origin',(80.,0.,28.));
#6741=CARTESIAN_POINT('',(80.,10.,28.));
#6742=CARTESIAN_POINT('',(80.,-10.,28.));
#6743=CARTESIAN_POINT('Origin',(80.,0.,28.));
#6744=CARTESIAN_POINT('',(80.,8.,30.));
#6745=CARTESIAN_POINT('Origin',(80.,8.,28.));
#6746=CARTESIAN_POINT('',(80.,-8.,30.));
#6747=CARTESIAN_POINT('Origin',(80.,0.,30.));
#6748=CARTESIAN_POINT('Origin',(80.,-8.,28.));
#6749=CARTESIAN_POINT('Origin',(80.,0.,-30.));
#6750=CARTESIAN_POINT('',(85.,6.12323399573677E-16,-30.));
#6751=CARTESIAN_POINT('Origin',(80.,0.,-30.));
#6752=CARTESIAN_POINT('',(85.,6.12323399573677E-16,-22.));
#6753=CARTESIAN_POINT('',(85.,6.12323399573677E-16,-30.));
#6754=CARTESIAN_POINT('Origin',(80.,0.,-22.));
#6755=CARTESIAN_POINT('Origin',(-10.352761804101,-38.6370330515627,-30.));
#6756=CARTESIAN_POINT('',(-0.693503541210314,-41.2252235025879,-5.));
#6757=CARTESIAN_POINT('',(-0.693503541210314,-41.2252235025879,-30.));
#6758=CARTESIAN_POINT('',(-20.0120200669917,-36.0488426005374,-5.));
#6759=CARTESIAN_POINT('Origin',(-10.352761804101,-38.6370330515627,-5.));
#6760=CARTESIAN_POINT('',(-20.0120200669917,-36.0488426005374,-30.));
#6761=CARTESIAN_POINT('Origin',(80.,0.,30.));
#6762=CARTESIAN_POINT('',(85.,-6.12323399573677E-16,30.));
#6763=CARTESIAN_POINT('Origin',(80.,0.,30.));
#6764=CARTESIAN_POINT('',(85.,-6.12323399573677E-16,22.));
#6765=CARTESIAN_POINT('',(85.,-6.12323399573677E-16,30.));
#6766=CARTESIAN_POINT('Origin',(80.,0.,22.));
#6767=CARTESIAN_POINT('Origin',(-10.352761804101,-38.6370330515627,30.));
#6768=CARTESIAN_POINT('',(-0.693503541210314,-41.2252235025879,8.));
#6769=CARTESIAN_POINT('',(-20.0120200669917,-36.0488426005374,8.));
#6770=CARTESIAN_POINT('Origin',(-10.352761804101,-38.6370330515627,8.));
#6771=CARTESIAN_POINT('',(-20.0120200669917,-36.0488426005374,5.));
#6772=CARTESIAN_POINT('',(-20.0120200669917,-36.0488426005374,30.));
#6773=CARTESIAN_POINT('',(-0.693503541210314,-41.2252235025879,5.));
#6774=CARTESIAN_POINT('Origin',(-10.352761804101,-38.6370330515627,5.));
#6775=CARTESIAN_POINT('',(-0.693503541210314,-41.2252235025879,30.));
#6776=CARTESIAN_POINT('Origin',(0.,0.,30.));
#6777=CARTESIAN_POINT('',(10.,-1.22464679914735E-15,-15.));
#6778=CARTESIAN_POINT('Origin',(0.,0.,-15.));
#6779=CARTESIAN_POINT('',(10.,-1.22464679914735E-15,-12.));
#6780=CARTESIAN_POINT('',(10.,-1.22464679914735E-15,30.));
#6781=CARTESIAN_POINT('',(-8.36862877099655,-5.47412572866653,-12.));
#6782=CARTESIAN_POINT('Origin',(0.,0.,-12.));
#6783=CARTESIAN_POINT('',(-10.0001237867953,1.97103394976209E-9,-9.76179717313037));
#6784=CARTESIAN_POINT('Ctrl Pts',(-8.36862877099655,-5.47412572866653,-12.));
#6785=CARTESIAN_POINT('Ctrl Pts',(-8.45441677353284,-5.3429763941761,-11.999999997427));
#6786=CARTESIAN_POINT('Ctrl Pts',(-8.53638588592189,-5.21097527038014,-11.9927750050672));
#6787=CARTESIAN_POINT('Ctrl Pts',(-8.61474990666338,-5.07804162738316,-11.9792446203911));
#6788=CARTESIAN_POINT('Ctrl Pts',(-8.69764757311686,-4.93741728609315,-11.9649314533886));
#6789=CARTESIAN_POINT('Ctrl Pts',(-8.7765110195439,-4.79574947320889,-11.9435619214423));
#6790=CARTESIAN_POINT('Ctrl Pts',(-8.85157147514725,-4.65293688559633,-11.9161702848848));
#6791=CARTESIAN_POINT('Ctrl Pts',(-8.88099655546167,-4.59695172234851,-11.9054322591271));
#6792=CARTESIAN_POINT('Ctrl Pts',(-8.90983696513968,-4.54079056665035,-11.8937682266929));
#6793=CARTESIAN_POINT('Ctrl Pts',(-8.93810575967581,-4.4844470594322,-11.8812385781177));
#6794=CARTESIAN_POINT('Ctrl Pts',(-9.00060480640978,-4.35987805857574,-11.8535369691632));
#6795=CARTESIAN_POINT('Ctrl Pts',(-9.06035407011131,-4.23417994539579,-11.8214303185381));
#6796=CARTESIAN_POINT('Ctrl Pts',(-9.11723772204825,-4.107888608141,-11.7855218310165));
#6797=CARTESIAN_POINT('Ctrl Pts',(-9.17291702662629,-3.9842711259095,-11.7503736022096));
#6798=CARTESIAN_POINT('Ctrl Pts',(-9.22565175869234,-3.86052975248589,-11.7117034479191));
#6799=CARTESIAN_POINT('Ctrl Pts',(-9.27540566403723,-3.73710738033695,-11.6701121216955));
#6800=CARTESIAN_POINT('Ctrl Pts',(-9.31297518633027,-3.64391028294799,-11.6387062200497));
#6801=CARTESIAN_POINT('Ctrl Pts',(-9.34884483253428,-3.55089436934357,-11.6056335296996));
#6802=CARTESIAN_POINT('Ctrl Pts',(-9.3829931498531,-3.45824226410632,-11.5711359915397));
#6803=CARTESIAN_POINT('Ctrl Pts',(-9.4344758472812,-3.31855806662537,-11.5191268016721));
#6804=CARTESIAN_POINT('Ctrl Pts',(-9.48228811673317,-3.17928629062166,-11.4637999274883));
#6805=CARTESIAN_POINT('Ctrl Pts',(-9.52668028722712,-3.04019414324163,-11.4054943378528));
#6806=CARTESIAN_POINT('Ctrl Pts',(-9.56112163353964,-2.93228050072395,-11.3602583653323));
#6807=CARTESIAN_POINT('Ctrl Pts',(-9.5935035091139,-2.8244750314983,-11.3132284064526));
#6808=CARTESIAN_POINT('Ctrl Pts',(-9.62392825897893,-2.71666946271822,-11.2645470181033));
#6809=CARTESIAN_POINT('Ctrl Pts',(-9.65106802401281,-2.62050374832403,-11.2211217985967));
#6810=CARTESIAN_POINT('Ctrl Pts',(-9.67662805956223,-2.52441492191825,-11.1764028555152));
#6811=CARTESIAN_POINT('Ctrl Pts',(-9.70066935863215,-2.42837682308185,-11.1305171637202));
#6812=CARTESIAN_POINT('Ctrl Pts',(-9.73425070221459,-2.29422898087712,-11.0664231571024));
#6813=CARTESIAN_POINT('Ctrl Pts',(-9.76488031347849,-2.16005590238908,-10.9999667510052));
#6814=CARTESIAN_POINT('Ctrl Pts',(-9.79262273697897,-2.02595889184267,-10.9314471311979));
#6815=CARTESIAN_POINT('Ctrl Pts',(-9.81788538848297,-1.90384821736955,-10.8690521758203));
#6816=CARTESIAN_POINT('Ctrl Pts',(-9.84075817492368,-1.78176050965276,-10.8049283493925));
#6817=CARTESIAN_POINT('Ctrl Pts',(-9.86124220206778,-1.66008483923076,-10.7394558128057));
#6818=CARTESIAN_POINT('Ctrl Pts',(-9.87618462610704,-1.57132643982444,-10.6916957508939));
#6819=CARTESIAN_POINT('Ctrl Pts',(-9.8898569179316,-1.48278733165533,-10.6432187826923));
#6820=CARTESIAN_POINT('Ctrl Pts',(-9.90227459651842,-1.39461744436331,-10.5941810273421));
#6821=CARTESIAN_POINT('Ctrl Pts',(-9.90491108546458,-1.37589744516181,-10.5837694597515));
#6822=CARTESIAN_POINT('Ctrl Pts',(-9.90749042320112,-1.35720601089956,-10.5733402505487));
#6823=CARTESIAN_POINT('Ctrl Pts',(-9.91001294263523,-1.33854404163214,-10.5628944871018));
#6824=CARTESIAN_POINT('Ctrl Pts',(-9.93626127877299,-1.1443549956723,-10.4542000182056));
#6825=CARTESIAN_POINT('Ctrl Pts',(-9.95656708456508,-0.951820837724888,
-10.3428183419215));
#6826=CARTESIAN_POINT('Ctrl Pts',(-9.97120936406249,-0.760674650770803,
-10.2291898572203));
#6827=CARTESIAN_POINT('Ctrl Pts',(-9.98607735096438,-0.566581988867939,
-10.1138098153001));
#6828=CARTESIAN_POINT('Ctrl Pts',(-9.99510564348261,-0.373919899057051,
-9.99611300520595));
#6829=CARTESIAN_POINT('Ctrl Pts',(-9.99856425937658,-0.182425776511984,
-9.876514630881));
#6830=CARTESIAN_POINT('Ctrl Pts',(-9.99966462607587,-0.121501475573082,
-9.83846412963148));
#6831=CARTESIAN_POINT('Ctrl Pts',(-10.0002010743077,-0.0606955535016998,
-9.80022081609969));
#6832=CARTESIAN_POINT('Ctrl Pts',(-10.0001819091909,-1.39135034132474E-8,
-9.76179714435925));
#6833=CARTESIAN_POINT('',(-9.65925826289068,2.58819045102525,-8.));
#6834=CARTESIAN_POINT('Ctrl Pts',(-10.,3.58012980029344E-8,-9.76179723440599));
#6835=CARTESIAN_POINT('Ctrl Pts',(-10.,0.441544717876623,-9.48226950053063));
#6836=CARTESIAN_POINT('Ctrl Pts',(-9.97097024786624,0.87720718112473,-9.19317827898892));
#6837=CARTESIAN_POINT('Ctrl Pts',(-9.85692793745532,1.7408939537672,-8.60247731152257));
#6838=CARTESIAN_POINT('Ctrl Pts',(-9.77133803228051,2.16990305716179,-8.30002077297609));
#6839=CARTESIAN_POINT('Ctrl Pts',(-9.65925826289068,2.58819045102525,-8.));
#6840=CARTESIAN_POINT('',(-9.65925826289068,2.58819045102525,8.));
#6841=CARTESIAN_POINT('',(-9.65925826289068,2.58819045102525,30.));
#6842=CARTESIAN_POINT('',(-10.0001237867953,1.97103495948311E-9,9.76179717313037));
#6843=CARTESIAN_POINT('Ctrl Pts',(-9.65925826289068,2.58819045102525,8.));
#6844=CARTESIAN_POINT('Ctrl Pts',(-9.77163928663693,2.16877876059763,8.30082718581888));
#6845=CARTESIAN_POINT('Ctrl Pts',(-9.85693279744154,1.74086457562841,8.60249771169349));
#6846=CARTESIAN_POINT('Ctrl Pts',(-9.97097123275185,0.877192293395072,9.1931881535409));
#6847=CARTESIAN_POINT('Ctrl Pts',(-10.,0.441537174494764,9.48227427600301));
#6848=CARTESIAN_POINT('Ctrl Pts',(-10.,3.58012987980397E-8,9.76179723440599));
#6849=CARTESIAN_POINT('Ctrl Pts',(-10.0001819091909,-1.39135025250588E-8,
9.76179714435925));
#6850=CARTESIAN_POINT('Ctrl Pts',(-10.0002422168267,-0.190993084247708,
9.88270644163236));
#6851=CARTESIAN_POINT('Ctrl Pts',(-9.99480220281986,-0.383077493992189,
10.00183306457));
#6852=CARTESIAN_POINT('Ctrl Pts',(-9.98359703547028,-0.576510028433417,
10.118774303758));
#6853=CARTESIAN_POINT('Ctrl Pts',(-9.97256127034954,-0.767018206509035,
10.2339475991086));
#6854=CARTESIAN_POINT('Ctrl Pts',(-9.95593360360136,-0.95883449076797,10.3470012231726));
#6855=CARTESIAN_POINT('Ctrl Pts',(-9.93344119546686,-1.15222238942891,10.4575076433073));
#6856=CARTESIAN_POINT('Ctrl Pts',(-9.9262367904895,-1.21416527839578,10.4929032754017));
#6857=CARTESIAN_POINT('Ctrl Pts',(-9.91843052664459,-1.27626951880198,10.5280372367801));
#6858=CARTESIAN_POINT('Ctrl Pts',(-9.91001294263524,-1.33854404163207,10.562894487102));
#6859=CARTESIAN_POINT('Ctrl Pts',(-9.90749042320113,-1.35720601089949,10.5733402505489));
#6860=CARTESIAN_POINT('Ctrl Pts',(-9.90491108546458,-1.37589744516174,10.5837694597516));
#6861=CARTESIAN_POINT('Ctrl Pts',(-9.90227459651842,-1.39461744436323,10.5941810273423));
#6862=CARTESIAN_POINT('Ctrl Pts',(-9.8852516513421,-1.51548634486515,10.6614051075165));
#6863=CARTESIAN_POINT('Ctrl Pts',(-9.86586922292159,-1.63704928825616,10.7275744442729));
#6864=CARTESIAN_POINT('Ctrl Pts',(-9.84409332992305,-1.75891940227426,10.7922898679902));
#6865=CARTESIAN_POINT('Ctrl Pts',(-9.82820853223256,-1.84781964190271,10.8394976409744));
#6866=CARTESIAN_POINT('Ctrl Pts',(-9.81105101031158,-1.93688317128088,10.8859320635458));
#6867=CARTESIAN_POINT('Ctrl Pts',(-9.79262273697897,-2.02595889184268,10.9314471311979));
#6868=CARTESIAN_POINT('Ctrl Pts',(-9.76488031347849,-2.16005590238909,10.9999667510052));
#6869=CARTESIAN_POINT('Ctrl Pts',(-9.73425070221459,-2.29422898087712,11.0664231571024));
#6870=CARTESIAN_POINT('Ctrl Pts',(-9.70066935863215,-2.42837682308185,11.1305171637201));
#6871=CARTESIAN_POINT('Ctrl Pts',(-9.67662805956223,-2.52441492191826,11.1764028555152));
#6872=CARTESIAN_POINT('Ctrl Pts',(-9.65106802401281,-2.62050374832403,11.2211217985967));
#6873=CARTESIAN_POINT('Ctrl Pts',(-9.62392825897893,-2.71666946271822,11.2645470181033));
#6874=CARTESIAN_POINT('Ctrl Pts',(-9.58471316352384,-2.85562231160131,11.3272934761505));
#6875=CARTESIAN_POINT('Ctrl Pts',(-9.5422477893575,-2.9945749698244,11.387297557256));
#6876=CARTESIAN_POINT('Ctrl Pts',(-9.49630917584708,-3.13375936775937,11.4442500498319));
#6877=CARTESIAN_POINT('Ctrl Pts',(-9.46066803283884,-3.24174458220626,11.488436231727));
#6878=CARTESIAN_POINT('Ctrl Pts',(-9.42293563050879,-3.34986928377481,11.5307850355101));
#6879=CARTESIAN_POINT('Ctrl Pts',(-9.3829931498531,-3.45824226410632,11.5711359915397));
#6880=CARTESIAN_POINT('Ctrl Pts',(-9.33776999970747,-3.58094289463323,11.6168216203012));
#6881=CARTESIAN_POINT('Ctrl Pts',(-9.28952854437317,-3.70428222851569,11.6600098053998));
#6882=CARTESIAN_POINT('Ctrl Pts',(-9.23831661995914,-3.82783387752058,11.7001335892842));
#6883=CARTESIAN_POINT('Ctrl Pts',(-9.19964613725768,-3.92112859276999,11.7304313394346));
#6884=CARTESIAN_POINT('Ctrl Pts',(-9.15928155479108,-4.01454418176179,11.7589811573433));
#6885=CARTESIAN_POINT('Ctrl Pts',(-9.11723772204827,-4.10788860814096,11.7855218310166));
#6886=CARTESIAN_POINT('Ctrl Pts',(-9.06035407011132,-4.23417994539576,11.8214303185383));
#6887=CARTESIAN_POINT('Ctrl Pts',(-9.00060480640979,-4.35987805857573,11.8535369691633));
#6888=CARTESIAN_POINT('Ctrl Pts',(-8.93810575967581,-4.4844470594322,11.8812385781177));
#6889=CARTESIAN_POINT('Ctrl Pts',(-8.8655173877299,-4.62912544157758,11.9134121039451));
#6890=CARTESIAN_POINT('Ctrl Pts',(-8.78916153683245,-4.7726019250157,11.9398813478119));
#6891=CARTESIAN_POINT('Ctrl Pts',(-8.70881072233522,-4.91498224698192,11.9596101136812));
#6892=CARTESIAN_POINT('Ctrl Pts',(-8.63305448011727,-5.04922106242435,11.9782107610451));
#6893=CARTESIAN_POINT('Ctrl Pts',(-8.55374701687845,-5.1824854269134,11.9908200299044));
#6894=CARTESIAN_POINT('Ctrl Pts',(-8.4706795483874,-5.31485894338431,11.9965268972474));
#6895=CARTESIAN_POINT('Ctrl Pts',(-8.4372756670212,-5.36809024223746,11.9988217970819));
#6896=CARTESIAN_POINT('Ctrl Pts',(-8.40326355436336,-5.42117742990113,11.9999999989612));
#6897=CARTESIAN_POINT('Ctrl Pts',(-8.36862877099654,-5.47412572866653,12.));
#6898=CARTESIAN_POINT('',(10.,-1.22464679914735E-15,15.));
#6899=CARTESIAN_POINT('',(10.,-1.22464679914735E-15,30.));
#6900=CARTESIAN_POINT('Origin',(0.,0.,15.));
#6901=CARTESIAN_POINT('',(0.,10.,8.));
#6902=CARTESIAN_POINT('Ctrl Pts',(7.4535599249993,6.66666666666667,12.));
#6903=CARTESIAN_POINT('Ctrl Pts',(7.32443309352201,6.81103485311786,11.99999999682));
#6904=CARTESIAN_POINT('Ctrl Pts',(7.19246919567612,6.9501822010365,11.9889588601183));
#6905=CARTESIAN_POINT('Ctrl Pts',(7.0576993924076,7.08444300037639,11.9685994397917));
#6906=CARTESIAN_POINT('Ctrl Pts',(6.92292958913909,7.21870379971628,11.9482400194651));
#6907=CARTESIAN_POINT('Ctrl Pts',(6.78535384384508,7.34807802019908,11.9185618083842));
#6908=CARTESIAN_POINT('Ctrl Pts',(6.64499605849823,7.47288614812075,11.8812318773614));
#6909=CARTESIAN_POINT('Ctrl Pts',(6.63654366979561,7.48040213170394,11.8789838575137));
#6910=CARTESIAN_POINT('Ctrl Pts',(6.62807974800606,7.48790223671562,11.8767069196995));
#6911=CARTESIAN_POINT('Ctrl Pts',(6.61960457791775,7.49538631823325,11.8744014042209));
#6912=CARTESIAN_POINT('Ctrl Pts',(6.48185055268487,7.61703135231309,11.8369279335891));
#6913=CARTESIAN_POINT('Ctrl Pts',(6.34120540493964,7.73437093825154,11.791921326457));
#6914=CARTESIAN_POINT('Ctrl Pts',(6.19898657325189,7.84672900130041,11.7408838129976));
#6915=CARTESIAN_POINT('Ctrl Pts',(6.05676774156413,7.95908706434928,11.6898462995382));
#6916=CARTESIAN_POINT('Ctrl Pts',(5.9129759592346,8.06646321098892,11.6327787221492));
#6917=CARTESIAN_POINT('Ctrl Pts',(5.76889672089669,8.16822077470328,11.571161743219));
#6918=CARTESIAN_POINT('Ctrl Pts',(5.75379442418606,8.1788869396379,11.5647030895716));
#6919=CARTESIAN_POINT('Ctrl Pts',(5.73868373288969,8.18949663728534,11.5581931861037));
#6920=CARTESIAN_POINT('Ctrl Pts',(5.72356470502882,8.2000502330104,11.5516328635545));
#6921=CARTESIAN_POINT('Ctrl Pts',(5.54237464595592,8.32652705747638,11.4730123833783));
#6922=CARTESIAN_POINT('Ctrl Pts',(5.35972864022817,8.44512957455917,11.3870622034709));
#6923=CARTESIAN_POINT('Ctrl Pts',(5.17553266659185,8.55653116699126,11.2950285747769));
#6924=CARTESIAN_POINT('Ctrl Pts',(5.06965587040675,8.6205653772065,11.2421271700663));
#6925=CARTESIAN_POINT('Ctrl Pts',(4.96326699017399,8.68221979432739,11.18721494629));
#6926=CARTESIAN_POINT('Ctrl Pts',(4.85634813127281,8.7416178610103,11.1305223120243));
#6927=CARTESIAN_POINT('Ctrl Pts',(4.83760485921073,8.75203056214872,11.1205838832113));
#6928=CARTESIAN_POINT('Ctrl Pts',(4.81884248159145,8.76237495465752,11.1105886554459));
#6929=CARTESIAN_POINT('Ctrl Pts',(4.80006143083322,8.77265117277875,11.1005377116491));
#6930=CARTESIAN_POINT('Ctrl Pts',(4.67853878586853,8.83914336335964,11.035503156858));
#6931=CARTESIAN_POINT('Ctrl Pts',(4.55611379988328,8.9028432066626,10.9680753730249));
#6932=CARTESIAN_POINT('Ctrl Pts',(4.43314656586013,8.96365874967832,10.8986785149911));
#6933=CARTESIAN_POINT('Ctrl Pts',(4.30539927968577,9.02683834901789,10.8265840228829));
#6934=CARTESIAN_POINT('Ctrl Pts',(4.17706707175951,9.08690480285482,10.7523650450191));
#6935=CARTESIAN_POINT('Ctrl Pts',(4.04856409267038,9.14380227472548,10.6765257027452));
#6936=CARTESIAN_POINT('Ctrl Pts',(4.0023909454348,9.16424643379976,10.6492754308691));
#6937=CARTESIAN_POINT('Ctrl Pts',(3.95619582194605,9.1842818998028,10.6218161673034));
#6938=CARTESIAN_POINT('Ctrl Pts',(3.90999812363261,9.2039075764655,10.5941718862756));
#6939=CARTESIAN_POINT('Ctrl Pts',(3.8904775206927,9.21220030652664,10.5824909356394));
#6940=CARTESIAN_POINT('Ctrl Pts',(3.87097075026249,9.22041521797258,10.5707865416166));
#6941=CARTESIAN_POINT('Ctrl Pts',(3.85147861510306,9.22855261214377,10.559059913264));
#6942=CARTESIAN_POINT('Ctrl Pts',(3.60036010696405,9.33338721685456,10.4079849595288));
#6943=CARTESIAN_POINT('Ctrl Pts',(3.34928636559173,9.42635559679678,10.2518372325069));
#6944=CARTESIAN_POINT('Ctrl Pts',(3.09786269543073,9.50831050937557,10.0916156638059));
#6945=CARTESIAN_POINT('Ctrl Pts',(2.83364682712233,9.59443521026502,9.92324217347811));
#6946=CARTESIAN_POINT('Ctrl Pts',(2.56904501266554,9.66839715764356,9.75036930809004));
#6947=CARTESIAN_POINT('Ctrl Pts',(2.30359960581663,9.73113308394545,9.57413333089425));
#6948=CARTESIAN_POINT('Ctrl Pts',(2.19421189175197,9.75698600658351,9.50150803701462));
#6949=CARTESIAN_POINT('Ctrl Pts',(2.08468088072785,9.7809319426623,9.42831140146962));
#6950=CARTESIAN_POINT('Ctrl Pts',(1.974974279851,9.80303405043287,9.35462218793377));
#6951=CARTESIAN_POINT('Ctrl Pts',(1.9634639600312,9.80535298408953,9.34689078063204));
#6952=CARTESIAN_POINT('Ctrl Pts',(1.9519511325459,9.80765144332111,9.33915328863826));
#6953=CARTESIAN_POINT('Ctrl Pts',(1.94043581192868,9.80992942994645,9.33140979991383));
#6954=CARTESIAN_POINT('Ctrl Pts',(1.76247768584885,9.84513350671991,9.21174168223595));
#6955=CARTESIAN_POINT('Ctrl Pts',(1.58405644832137,9.87542603772905,9.09072486559958));
#6956=CARTESIAN_POINT('Ctrl Pts',(1.40504595874219,9.90084697353231,8.96857634820572));
#6957=CARTESIAN_POINT('Ctrl Pts',(1.26163873401112,9.92121195807696,8.87072185975843));
#6958=CARTESIAN_POINT('Ctrl Pts',(1.11785322956714,9.93844951919808,8.77214041219644));
#6959=CARTESIAN_POINT('Ctrl Pts',(0.973624298149134,9.95255818426511,8.67293388154916));
#6960=CARTESIAN_POINT('Ctrl Pts',(0.82272776139333,9.96731908331589,8.56914110050965));
#6961=CARTESIAN_POINT('Ctrl Pts',(0.671530069329876,9.97863100442017,8.46479064327355));
#6962=CARTESIAN_POINT('Ctrl Pts',(0.520367904445434,9.98649236040718,8.36027671301796));
#6963=CARTESIAN_POINT('Ctrl Pts',(0.368186462519023,9.99440672502689,8.25505805185462));
#6964=CARTESIAN_POINT('Ctrl Pts',(0.216041172145373,9.99882382364899,8.14967421046749));
#6965=CARTESIAN_POINT('Ctrl Pts',(0.0642766288123017,9.99979448577473,8.04453172419152));
#6966=CARTESIAN_POINT('Ctrl Pts',(0.0428431687350635,9.99993157081095,8.02968262154525));
#6967=CARTESIAN_POINT('Ctrl Pts',(0.0214173025071013,10.,8.01483833249367));
#6968=CARTESIAN_POINT('Ctrl Pts',(1.33226762955019E-15,10.,8.));
#6969=CARTESIAN_POINT('',(0.,10.,-8.));
#6970=CARTESIAN_POINT('',(0.,10.,30.));
#6971=CARTESIAN_POINT('',(7.4535599249993,6.66666666666667,-12.));
#6972=CARTESIAN_POINT('Ctrl Pts',(0.,10.,-8.));
#6973=CARTESIAN_POINT('Ctrl Pts',(0.209085099686919,10.,-8.14485830919264));
#6974=CARTESIAN_POINT('Ctrl Pts',(0.418288781390105,9.99347420733504,-8.28980641296881));
#6975=CARTESIAN_POINT('Ctrl Pts',(0.627262534901026,9.98035857777825,-8.43416422574658));
#6976=CARTESIAN_POINT('Ctrl Pts',(0.847178419334319,9.96655619721408,-8.58608079679203));
#6977=CARTESIAN_POINT('Ctrl Pts',(1.06683943516283,9.94545528423446,-8.73734285597004));
#6978=CARTESIAN_POINT('Ctrl Pts',(1.28584122492737,9.91704302479201,-8.88715246988158));
#6979=CARTESIAN_POINT('Ctrl Pts',(1.49281407510468,9.89019134324591,-9.02873360859543));
#6980=CARTESIAN_POINT('Ctrl Pts',(1.69919797291203,9.85680994096409,-9.16901679075694));
#6981=CARTESIAN_POINT('Ctrl Pts',(1.90465594999555,9.81694004719906,-9.30733474421298));
#6982=CARTESIAN_POINT('Ctrl Pts',(1.91659684751875,9.814622871091,-9.31537356816755));
#6983=CARTESIAN_POINT('Ctrl Pts',(1.9285346191681,9.81228379261445,-9.32340575754666));
#6984=CARTESIAN_POINT('Ctrl Pts',(1.94046919944125,9.80992282509999,-9.33143118277434));
#6985=CARTESIAN_POINT('Ctrl Pts',(1.95197352173875,9.80764697370023,-9.33916728042341));
#6986=CARTESIAN_POINT('Ctrl Pts',(1.96347535561302,9.80535068876919,-9.34689739267515));
#6987=CARTESIAN_POINT('Ctrl Pts',(1.97497468657832,9.80303396849238,-9.35462143181174));
#6988=CARTESIAN_POINT('Ctrl Pts',(2.24251254824573,9.74913427721365,-9.53432518329739));
#6989=CARTESIAN_POINT('Ctrl Pts',(2.5090065924052,9.68427253191354,-9.71110047463118));
#6990=CARTESIAN_POINT('Ctrl Pts',(2.7749232834884,9.60751844470339,-9.88380087138435));
#6991=CARTESIAN_POINT('Ctrl Pts',(3.02784790867845,9.5345143821891,-10.0480635317726));
#6992=CARTESIAN_POINT('Ctrl Pts',(3.28024979088569,9.45075168409379,-10.2086402039897));
#6993=CARTESIAN_POINT('Ctrl Pts',(3.53252798197937,9.35538605373282,-10.3645278522479));
#6994=CARTESIAN_POINT('Ctrl Pts',(3.6388640692924,9.31518912686901,-10.4302350087181));
#6995=CARTESIAN_POINT('Ctrl Pts',(3.74517818821727,9.2729302095569,-10.4951088432616));
#6996=CARTESIAN_POINT('Ctrl Pts',(3.85150038699593,9.22854352298752,-10.5590730208312));
#6997=CARTESIAN_POINT('Ctrl Pts',(3.87098527378687,9.22040910164594,-10.5707952648493));
#6998=CARTESIAN_POINT('Ctrl Pts',(3.89048478576427,9.21219722017683,-10.5824952913507));
#6999=CARTESIAN_POINT('Ctrl Pts',(3.9099981209759,9.20390757759402,-10.5941718925655));
#7000=CARTESIAN_POINT('Ctrl Pts',(4.03898075658645,9.14911325683834,-10.6713539213333));
#7001=CARTESIAN_POINT('Ctrl Pts',(4.16794297285713,9.09112109034215,-10.7470924847379));
#7002=CARTESIAN_POINT('Ctrl Pts',(4.29646417587719,9.02997028952467,-10.8208712485592));
#7003=CARTESIAN_POINT('Ctrl Pts',(4.42014485896863,8.97112262362231,-10.8918712679539));
#7004=CARTESIAN_POINT('Ctrl Pts',(4.54341682842248,8.90934998996412,-10.9610556950588));
#7005=CARTESIAN_POINT('Ctrl Pts',(4.66591280664953,8.84472972017589,-11.0279859964137));
#7006=CARTESIAN_POINT('Ctrl Pts',(4.71074408320321,8.82107988915467,-11.0524812565299));
#7007=CARTESIAN_POINT('Ctrl Pts',(4.75547151809011,8.79704904424051,-11.0766748545963));
#7008=CARTESIAN_POINT('Ctrl Pts',(4.80007749004456,8.77264238582005,-11.1005463067514));
#7009=CARTESIAN_POINT('Ctrl Pts',(4.81885317713414,8.76236905780305,-11.1105943540508));
#7010=CARTESIAN_POINT('Ctrl Pts',(4.8376102014733,8.7520275942893,-11.1205867167142));
#7011=CARTESIAN_POINT('Ctrl Pts',(4.85634813102705,8.74161786114682,-11.1305223127522));
#7012=CARTESIAN_POINT('Ctrl Pts',(5.04235190637572,8.63828469088813,-11.229148917581));
#7013=CARTESIAN_POINT('Ctrl Pts',(5.22675176126298,8.5281243719752,-11.32238944137));
#7014=CARTESIAN_POINT('Ctrl Pts',(5.40964172666946,8.41048088884993,-11.40902216654));
#7015=CARTESIAN_POINT('Ctrl Pts',(5.51477922677033,8.34285147194091,-11.4588245060564));
#7016=CARTESIAN_POINT('Ctrl Pts',(5.61941772167317,8.27274856573666,-11.5064424239632));
#7017=CARTESIAN_POINT('Ctrl Pts',(5.72357511243166,8.20004296827939,-11.5516373819622));
#7018=CARTESIAN_POINT('Ctrl Pts',(5.73869066712922,8.18949176853081,-11.5581961758674));
#7019=CARTESIAN_POINT('Ctrl Pts',(5.75379788912304,8.17888449248633,-11.5647045736646));
#7020=CARTESIAN_POINT('Ctrl Pts',(5.76889672042948,8.16822077503325,-11.5711617451841));
#7021=CARTESIAN_POINT('Ctrl Pts',(5.91297681932932,8.06646260354981,-11.6327790910746));
#7022=CARTESIAN_POINT('Ctrl Pts',(6.05676946305485,7.95908577894731,-11.6898469834438));
#7023=CARTESIAN_POINT('Ctrl Pts',(6.19898913169897,7.84672698003327,-11.740884731588));
#7024=CARTESIAN_POINT('Ctrl Pts',(6.34120880034308,7.73436818111923,-11.7919224797322));
#7025=CARTESIAN_POINT('Ctrl Pts',(6.48185476056317,7.61702780143568,-11.8369292412042));
#7026=CARTESIAN_POINT('Ctrl Pts',(6.61960954778086,7.49538192954424,-11.874402757394));
#7027=CARTESIAN_POINT('Ctrl Pts',(6.62808305681875,7.48789930468805,-11.8767078110661));
#7028=CARTESIAN_POINT('Ctrl Pts',(6.63654532187993,7.48040066264689,-11.8789842981708));
#7029=CARTESIAN_POINT('Ctrl Pts',(6.64499605834415,7.47288614825776,-11.8812318786062));
#7030=CARTESIAN_POINT('Ctrl Pts',(6.78535384876212,7.34807801583195,-11.9185618113333));
#7031=CARTESIAN_POINT('Ctrl Pts',(6.92292959388377,7.21870379512185,-11.9482400216728));
#7032=CARTESIAN_POINT('Ctrl Pts',(7.05769939588734,7.08444299690985,-11.9685994412462));
#7033=CARTESIAN_POINT('Ctrl Pts',(7.1924691978909,6.95018219869785,-11.9889588608196));
#7034=CARTESIAN_POINT('Ctrl Pts',(7.32443309337662,6.8110348532804,-11.99999999682));
#7035=CARTESIAN_POINT('Ctrl Pts',(7.4535599249993,6.66666666666667,-12.));
#7036=CARTESIAN_POINT('Origin',(0.,0.,-12.));
#7037=CARTESIAN_POINT('Origin',(0.,0.,10.));
#7038=CARTESIAN_POINT('',(-18.0801684144135,-36.5664806907425,10.));
#7039=CARTESIAN_POINT('',(-18.0801684144135,-36.5664806907425,10.));
#7040=CARTESIAN_POINT('',(-2.62535519378845,-40.7075854123829,10.));
#7041=CARTESIAN_POINT('Origin',(-10.352761804101,-38.6370330515627,10.));
#7042=CARTESIAN_POINT('',(1.76944146100923,-24.3059810077445,10.));
#7043=CARTESIAN_POINT('',(1.76944146100923,-24.3059810077445,10.));
#7044=CARTESIAN_POINT('',(23.0198096393687,-8.,10.));
#7045=CARTESIAN_POINT('Origin',(23.0198096393687,-30.,10.));
#7046=CARTESIAN_POINT('',(45.,-8.,10.));
#7047=CARTESIAN_POINT('',(47.,-8.,10.));
#7048=CARTESIAN_POINT('',(45.,8.,10.));
#7049=CARTESIAN_POINT('',(45.,1.56125112837913E-14,10.));
#7050=CARTESIAN_POINT('',(3.69090101271661E-16,8.,10.));
#7051=CARTESIAN_POINT('Origin',(-9.65925826289068,2.58819045102525,30.));
#7052=CARTESIAN_POINT('',(-9.65925826289068,2.58819045102525,8.));
#7053=CARTESIAN_POINT('',(-20.0120200669917,-36.0488426005374,-8.));
#7054=CARTESIAN_POINT('',(-15.8709153453513,-20.5940293799124,-5.));
#7055=CARTESIAN_POINT('',(-15.8709153453513,-20.5940293799124,-5.));
#7056=CARTESIAN_POINT('',(-15.8709153453513,-20.5940293799124,5.));
#7057=CARTESIAN_POINT('',(-15.8709153453513,-20.5940293799124,5.));
#7058=CARTESIAN_POINT('',(-15.8709153453513,-20.5940293799124,5.));
#7059=CARTESIAN_POINT('Origin',(-0.693503541210314,-41.2252235025879,30.));
#7060=CARTESIAN_POINT('',(3.70129311358736,-24.8236190979495,8.));
#7061=CARTESIAN_POINT('',(3.70129311358736,-24.8236190979495,-8.));
#7062=CARTESIAN_POINT('',(3.70129311358736,-24.8236190979495,30.));
#7063=CARTESIAN_POINT('',(-0.693503541210312,-41.2252235025879,8.));
#7064=CARTESIAN_POINT('',(3.44760118043008,-25.7704102819629,5.));
#7065=CARTESIAN_POINT('',(-0.693503541210314,-41.2252235025879,5.));
#7066=CARTESIAN_POINT('',(3.44760118043008,-25.7704102819629,-5.));
#7067=CARTESIAN_POINT('',(3.44760118043008,-25.7704102819629,5.));
#7068=CARTESIAN_POINT('',(-0.693503541210314,-41.2252235025879,-5.));
#7069=CARTESIAN_POINT('',(3.70129311358736,-24.8236190979495,-8.));
#7070=CARTESIAN_POINT('Origin',(23.0198096393687,-30.,30.));
#7071=CARTESIAN_POINT('',(23.0198096393687,-10.,8.));
#7072=CARTESIAN_POINT('',(23.0198096393687,-10.,-8.));
#7073=CARTESIAN_POINT('',(23.0198096393687,-10.,30.));
#7074=CARTESIAN_POINT('Origin',(23.0198096393687,-30.,8.));
#7075=CARTESIAN_POINT('Origin',(23.0198096393687,-30.,-8.));
#7076=CARTESIAN_POINT('Origin',(23.0198096393687,-10.,30.));
#7077=CARTESIAN_POINT('',(80.,-10.,22.));
#7078=CARTESIAN_POINT('',(80.,-10.,30.));
#7079=CARTESIAN_POINT('',(54.,-10.,28.));
#7080=CARTESIAN_POINT('',(54.,-10.,28.));
#7081=CARTESIAN_POINT('',(49.,-10.,23.));
#7082=CARTESIAN_POINT('Origin',(54.,-10.,23.));
#7083=CARTESIAN_POINT('',(49.,-10.,12.));
#7084=CARTESIAN_POINT('',(49.,-10.,30.));
#7085=CARTESIAN_POINT('',(45.,-10.,8.));
#7086=CARTESIAN_POINT('Origin',(45.,-10.,12.));
#7087=CARTESIAN_POINT('',(23.0198096393687,-10.,8.));
#7088=CARTESIAN_POINT('',(45.,-10.,-8.));
#7089=CARTESIAN_POINT('',(47.,-10.,-8.));
#7090=CARTESIAN_POINT('',(49.,-10.,-12.));
#7091=CARTESIAN_POINT('Origin',(45.,-10.,-12.));
#7092=CARTESIAN_POINT('',(49.,-10.,-23.));
#7093=CARTESIAN_POINT('',(49.,-10.,30.));
#7094=CARTESIAN_POINT('',(54.,-10.,-28.));
#7095=CARTESIAN_POINT('Origin',(54.,-10.,-23.));
#7096=CARTESIAN_POINT('',(80.,-10.,-28.));
#7097=CARTESIAN_POINT('',(80.,-10.,-28.));
#7098=CARTESIAN_POINT('',(80.,-10.,-22.));
#7099=CARTESIAN_POINT('',(80.,-10.,-30.));
#7100=CARTESIAN_POINT('',(54.,-10.,-22.));
#7101=CARTESIAN_POINT('',(54.,-10.,-22.));
#7102=CARTESIAN_POINT('',(54.,-10.,22.));
#7103=CARTESIAN_POINT('',(54.,-10.,22.));
#7104=CARTESIAN_POINT('',(54.,-10.,22.));
#7105=CARTESIAN_POINT('Origin',(0.,10.,30.));
#7106=CARTESIAN_POINT('',(49.,10.,23.));
#7107=CARTESIAN_POINT('',(54.,10.,28.));
#7108=CARTESIAN_POINT('Origin',(54.,10.,23.));
#7109=CARTESIAN_POINT('',(80.,10.,28.));
#7110=CARTESIAN_POINT('',(80.,10.,22.));
#7111=CARTESIAN_POINT('',(80.,10.,30.));
#7112=CARTESIAN_POINT('',(54.,10.,22.));
#7113=CARTESIAN_POINT('',(80.,10.,22.));
#7114=CARTESIAN_POINT('',(54.,10.,-22.));
#7115=CARTESIAN_POINT('',(54.,10.,22.));
#7116=CARTESIAN_POINT('',(80.,10.,-22.));
#7117=CARTESIAN_POINT('',(80.,10.,-22.));
#7118=CARTESIAN_POINT('',(80.,10.,-28.));
#7119=CARTESIAN_POINT('',(80.,10.,-30.));
#7120=CARTESIAN_POINT('',(54.,10.,-28.));
#7121=CARTESIAN_POINT('',(54.,10.,-28.));
#7122=CARTESIAN_POINT('',(49.,10.,-23.));
#7123=CARTESIAN_POINT('Origin',(54.,10.,-23.));
#7124=CARTESIAN_POINT('',(49.,10.,-12.));
#7125=CARTESIAN_POINT('',(49.,10.,30.));
#7126=CARTESIAN_POINT('',(45.,10.,-8.));
#7127=CARTESIAN_POINT('Origin',(45.,10.,-12.));
#7128=CARTESIAN_POINT('',(3.69090101271661E-16,10.,-8.));
#7129=CARTESIAN_POINT('',(45.,10.,8.));
#7130=CARTESIAN_POINT('',(47.,10.,8.));
#7131=CARTESIAN_POINT('',(49.,10.,12.));
#7132=CARTESIAN_POINT('Origin',(45.,10.,12.));
#7133=CARTESIAN_POINT('',(49.,10.,30.));
#7134=CARTESIAN_POINT('Origin',(0.,0.,30.));
#7135=CARTESIAN_POINT('',(54.,8.,30.));
#7136=CARTESIAN_POINT('',(54.,-8.,30.));
#7137=CARTESIAN_POINT('',(54.,-10.,30.));
#7138=CARTESIAN_POINT('',(80.,-8.,30.));
#7139=CARTESIAN_POINT('',(54.,8.,30.));
#7140=CARTESIAN_POINT('Origin',(80.,0.,30.));
#7141=CARTESIAN_POINT('Origin',(80.,0.,22.));
#7142=CARTESIAN_POINT('Origin',(54.,10.,22.));
#7143=CARTESIAN_POINT('',(54.,10.,-22.));
#7144=CARTESIAN_POINT('',(54.,10.,22.));
#7145=CARTESIAN_POINT('Origin',(80.,0.,22.));
#7146=CARTESIAN_POINT('Origin',(-15.8709153453513,-20.5940293799124,5.));
#7147=CARTESIAN_POINT('',(-15.8709153453513,-20.5940293799124,-5.));
#7148=CARTESIAN_POINT('',(-15.8709153453513,-20.5940293799124,5.));
#7149=CARTESIAN_POINT('Origin',(-10.352761804101,-38.6370330515627,5.));
#7150=CARTESIAN_POINT('Origin',(47.,10.,10.));
#7151=CARTESIAN_POINT('',(47.,-8.,23.));
#7152=CARTESIAN_POINT('',(47.,8.,23.));
#7153=CARTESIAN_POINT('',(47.,10.,23.));
#7154=CARTESIAN_POINT('',(47.,8.,12.));
#7155=CARTESIAN_POINT('',(47.,8.,10.));
#7156=CARTESIAN_POINT('',(47.,-8.,12.));
#7157=CARTESIAN_POINT('',(47.,10.,12.));
#7158=CARTESIAN_POINT('',(47.,-8.,10.));
#7159=CARTESIAN_POINT('Origin',(0.,0.,15.));
#7160=CARTESIAN_POINT('Origin',(0.,0.,-10.));
#7161=CARTESIAN_POINT('',(1.76944146100923,-24.3059810077445,-10.));
#7162=CARTESIAN_POINT('',(-2.62535519378845,-40.7075854123829,-10.));
#7163=CARTESIAN_POINT('',(-10.0423545251959,-6.56895087439983,-10.));
#7164=CARTESIAN_POINT('',(-7.72740661031254,2.0705523608202,-10.));
#7165=CARTESIAN_POINT('',(8.94427190999916,8.,-10.));
#7166=CARTESIAN_POINT('Origin',(0.,0.,-10.));
#7167=CARTESIAN_POINT('',(45.,8.,-10.));
#7168=CARTESIAN_POINT('',(47.,8.,-10.));
#7169=CARTESIAN_POINT('',(45.,-8.,-10.));
#7170=CARTESIAN_POINT('',(45.,1.56125112837913E-14,-10.));
#7171=CARTESIAN_POINT('',(23.0198096393687,-8.,-10.));
#7172=CARTESIAN_POINT('',(23.0198096393687,-8.,-10.));
#7173=CARTESIAN_POINT('Origin',(23.0198096393687,-30.,-10.));
#7174=CARTESIAN_POINT('Origin',(0.,0.,-30.));
#7175=CARTESIAN_POINT('',(80.,8.,-30.));
#7176=CARTESIAN_POINT('',(80.,-8.,-30.));
#7177=CARTESIAN_POINT('Origin',(80.,0.,-30.));
#7178=CARTESIAN_POINT('',(54.,-8.,-30.));
#7179=CARTESIAN_POINT('',(54.,-8.,-30.));
#7180=CARTESIAN_POINT('',(54.,8.,-30.));
#7181=CARTESIAN_POINT('',(54.,10.,-30.));
#7182=CARTESIAN_POINT('',(80.,8.,-30.));
#7183=CARTESIAN_POINT('Origin',(80.,0.,-30.));
#7184=CARTESIAN_POINT('Origin',(80.,0.,-28.));
#7185=CARTESIAN_POINT('Origin',(80.,0.,-22.));
#7186=CARTESIAN_POINT('Origin',(80.,0.,-22.));
#7187=CARTESIAN_POINT('Origin',(-10.352761804101,-38.6370330515627,-5.));
#7188=CARTESIAN_POINT('Origin',(47.,10.,-10.));
#7189=CARTESIAN_POINT('',(47.,8.,-23.));
#7190=CARTESIAN_POINT('',(47.,-8.,-23.));
#7191=CARTESIAN_POINT('',(47.,-10.,-23.));
#7192=CARTESIAN_POINT('',(47.,-8.,-12.));
#7193=CARTESIAN_POINT('',(47.,-8.,-10.));
#7194=CARTESIAN_POINT('',(47.,8.,-12.));
#7195=CARTESIAN_POINT('',(47.,10.,-12.));
#7196=CARTESIAN_POINT('',(47.,8.,-10.));
#7197=CARTESIAN_POINT('Origin',(0.,0.,-15.));
#7198=CARTESIAN_POINT('Origin',(54.,1.87350135405495E-14,-23.));
#7199=CARTESIAN_POINT('Origin',(54.,-8.,-23.));
#7200=CARTESIAN_POINT('Origin',(54.,8.,-23.));
#7201=CARTESIAN_POINT('Origin',(54.,10.,23.));
#7202=CARTESIAN_POINT('Origin',(54.,8.,23.));
#7203=CARTESIAN_POINT('Origin',(54.,-8.,23.));
#7204=CARTESIAN_POINT('Origin',(0.,8.,28.));
#7205=CARTESIAN_POINT('Origin',(54.,8.,28.));
#7206=CARTESIAN_POINT('Origin',(-4.8710921181488E-16,-8.,28.));
#7207=CARTESIAN_POINT('Origin',(54.,-8.,28.));
#7208=CARTESIAN_POINT('Origin',(54.,8.,23.));
#7209=CARTESIAN_POINT('Origin',(49.,8.,23.));
#7210=CARTESIAN_POINT('Origin',(54.,-8.,23.));
#7211=CARTESIAN_POINT('Origin',(49.,-8.,23.));
#7212=CARTESIAN_POINT('Origin',(49.,8.,30.));
#7213=CARTESIAN_POINT('Origin',(49.,8.,12.));
#7214=CARTESIAN_POINT('Origin',(45.,1.56125112837913E-14,12.));
#7215=CARTESIAN_POINT('Origin',(45.,-8.,12.));
#7216=CARTESIAN_POINT('Origin',(45.,8.,12.));
#7217=CARTESIAN_POINT('Origin',(49.,-8.,10.));
#7218=CARTESIAN_POINT('Origin',(49.,-8.,12.));
#7219=CARTESIAN_POINT('Origin',(45.,8.,12.));
#7220=CARTESIAN_POINT('Origin',(45.,8.,8.));
#7221=CARTESIAN_POINT('Origin',(45.,-8.,12.));
#7222=CARTESIAN_POINT('Origin',(45.,-8.,8.));
#7223=CARTESIAN_POINT('Origin',(0.,8.,8.));
#7224=CARTESIAN_POINT('Ctrl Pts',(8.94427190999916,8.,10.));
#7225=CARTESIAN_POINT('Ctrl Pts',(8.59397428869209,8.19582232339978,10.));
#7226=CARTESIAN_POINT('Ctrl Pts',(8.23809574830832,8.36927906280638,9.97233221567645));
#7227=CARTESIAN_POINT('Ctrl Pts',(7.51670439182639,8.68315531343203,9.88673268190064));
#7228=CARTESIAN_POINT('Ctrl Pts',(7.15119134028659,8.82341656046842,9.82830572643859));
#7229=CARTESIAN_POINT('Ctrl Pts',(6.41157022806713,9.07672862331535,9.69155908354252));
#7230=CARTESIAN_POINT('Ctrl Pts',(6.03624395121828,9.18999945289011,9.61279798983037));
#7231=CARTESIAN_POINT('Ctrl Pts',(5.28680518772518,9.39050807507187,9.44350384379107));
#7232=CARTESIAN_POINT('Ctrl Pts',(4.91193913605487,9.47807443933602,9.35282484136955));
#7233=CARTESIAN_POINT('Ctrl Pts',(3.78601706885828,9.70796487519961,9.06874336660609));
#7234=CARTESIAN_POINT('Ctrl Pts',(3.03362219917569,9.81784991817562,8.86354442007235));
#7235=CARTESIAN_POINT('Ctrl Pts',(1.90012638124304,9.92742805349748,8.54552077981019));
#7236=CARTESIAN_POINT('Ctrl Pts',(1.52148656713009,9.95463063545181,8.4377136379673));
#7237=CARTESIAN_POINT('Ctrl Pts',(0.762253747142684,9.99091801432738,8.22004456397749));
#7238=CARTESIAN_POINT('Ctrl Pts',(0.380054916719888,10.,8.10971233032629));
#7239=CARTESIAN_POINT('Ctrl Pts',(0.,10.,8.));
#7240=CARTESIAN_POINT('Origin',(-4.8710921181488E-16,-8.,8.));
#7241=CARTESIAN_POINT('Origin',(23.0198096393687,-8.,8.));
#7242=CARTESIAN_POINT('Ctrl Pts',(7.46595409979742,6.65278372912403,11.9999659823065));
#7243=CARTESIAN_POINT('Ctrl Pts',(7.46181137603258,6.65743228755678,9.99435834176235));
#7244=CARTESIAN_POINT('Ctrl Pts',(8.95919248103908,7.99171094663393,9.99998316436123));
#7245=CARTESIAN_POINT('Ctrl Pts',(7.2050090532042,6.94561778375818,12.0014006149718));
#7246=CARTESIAN_POINT('Ctrl Pts',(7.29338961739188,6.84609954078222,10.1091476443099));
#7247=CARTESIAN_POINT('Ctrl Pts',(8.64603010975786,8.16742618260248,10.0006968502176));
#7248=CARTESIAN_POINT('Ctrl Pts',(6.93129022829302,7.21830937991486,11.9573878676915));
#7249=CARTESIAN_POINT('Ctrl Pts',(7.08968233035302,7.06312387610362,10.1923050700163));
#7250=CARTESIAN_POINT('Ctrl Pts',(8.31758857577122,8.33102724263676,9.97868692248085));
#7251=CARTESIAN_POINT('Ctrl Pts',(6.36322946527443,7.7234369320712,11.8062939832124));
#7252=CARTESIAN_POINT('Ctrl Pts',(6.62330289734465,7.50555955075384,10.2799383797216));
#7253=CARTESIAN_POINT('Ctrl Pts',(7.63591040831743,8.63410122162527,9.90313394764094));
#7254=CARTESIAN_POINT('Ctrl Pts',(6.0676798404454,7.95720201860455,11.6989395444534));
#7255=CARTESIAN_POINT('Ctrl Pts',(6.36270324053587,7.73143421140555,10.2890080329594));
#7256=CARTESIAN_POINT('Ctrl Pts',(7.28124840537636,8.77435822208396,9.8494541734595));
#7257=CARTESIAN_POINT('Ctrl Pts',(5.47010836911268,8.37924322604346,11.4434059485407));
#7258=CARTESIAN_POINT('Ctrl Pts',(5.80819530329405,8.15710830657298,10.2436830242621));
#7259=CARTESIAN_POINT('Ctrl Pts',(6.56415809876884,9.02757824037212,9.72168360055666));
#7260=CARTESIAN_POINT('Ctrl Pts',(5.16605083626499,8.56956461250842,11.2947420399208));
#7261=CARTESIAN_POINT('Ctrl Pts',(5.51310144140328,8.36060172136931,10.1925886394282));
#7262=CARTESIAN_POINT('Ctrl Pts',(6.19928698920683,9.14176835009192,9.64735037171788));
#7263=CARTESIAN_POINT('Ctrl Pts',(4.54664343995125,8.91367221299836,10.9663084668338));
#7264=CARTESIAN_POINT('Ctrl Pts',(4.89532112501463,8.73555397522188,10.0437605916743));
#7265=CARTESIAN_POINT('Ctrl Pts',(5.45599414260708,9.34822738370456,9.48313222005185));
#7266=CARTESIAN_POINT('Ctrl Pts',(4.23052411852774,9.06774230389022,10.7859725905476));
#7267=CARTESIAN_POINT('Ctrl Pts',(4.5709050130387,8.9097084091423,9.94694323658702));
#7268=CARTESIAN_POINT('Ctrl Pts',(5.07664912268078,9.44066656892447,9.39296418997048));
#7269=CARTESIAN_POINT('Ctrl Pts',(3.26891873105192,9.47624976235846,10.2106353565519));
#7270=CARTESIAN_POINT('Ctrl Pts',(3.58252292320737,9.36878727249013,9.60992785891922));
#7271=CARTESIAN_POINT('Ctrl Pts',(3.92271663488453,9.68576304806697,9.1052966773183));
#7272=CARTESIAN_POINT('Ctrl Pts',(2.62559783884422,9.67195583771219,9.79164439618922));
#7273=CARTESIAN_POINT('Ctrl Pts',(2.88161358543654,9.60711253457495,9.32052272371477));
#7274=CARTESIAN_POINT('Ctrl Pts',(3.1507288339645,9.80318182826186,8.89580416339016));
#7275=CARTESIAN_POINT('Ctrl Pts',(1.32434891203353,9.93411262756739,8.91760334235447));
#7276=CARTESIAN_POINT('Ctrl Pts',(1.46612043782459,9.9184689874319,8.69236195992552));
#7277=CARTESIAN_POINT('Ctrl Pts',(1.58922406203033,9.96046940770512,8.45879148701049));
#7278=CARTESIAN_POINT('Ctrl Pts',(0.664585080193226,10.,8.46043776212904));
#7279=CARTESIAN_POINT('Ctrl Pts',(0.731002622520191,10.,8.34530575506384));
#7280=CARTESIAN_POINT('Ctrl Pts',(0.79752291803651,10.,8.23021899751621));
#7281=CARTESIAN_POINT('Ctrl Pts',(1.07753648825376E-35,10.,8.));
#7282=CARTESIAN_POINT('Ctrl Pts',(1.07753648825376E-35,10.,8.));
#7283=CARTESIAN_POINT('Ctrl Pts',(1.07753648825376E-35,10.,8.));
#7284=CARTESIAN_POINT('Origin',(23.0198096393687,-30.,8.));
#7285=CARTESIAN_POINT('Origin',(1.76944146100923,-24.3059810077445,8.));
#7286=CARTESIAN_POINT('Origin',(7.72740661031253,-2.07055236082019,8.));
#7287=CARTESIAN_POINT('Origin',(-2.62535519378845,-40.7075854123829,8.));
#7288=CARTESIAN_POINT('Ctrl Pts',(-10.038209642496,-6.58550840389661,9.99998316436182));
#7289=CARTESIAN_POINT('Ctrl Pts',(-8.36174489807087,-5.48442051636901,9.99435800706184));
#7290=CARTESIAN_POINT('Ctrl Pts',(-8.35842653183974,-5.48969106142489,12.0000850216378));
#7291=CARTESIAN_POINT('Ctrl Pts',(-10.1268851410615,-6.23753833216136,10.0006968502054));
#7292=CARTESIAN_POINT('Ctrl Pts',(-8.50039843904348,-5.27291666647825,10.1091539159912));
#7293=CARTESIAN_POINT('Ctrl Pts',(-8.57374963798823,-5.1618393734599,12.0015162133387));
#7294=CARTESIAN_POINT('Ctrl Pts',(-10.1999047059325,-5.87794510201831,9.97868692247048));
#7295=CARTESIAN_POINT('Ctrl Pts',(-8.6573118794847,-5.01998806659582,10.1923170765812));
#7296=CARTESIAN_POINT('Ctrl Pts',(-8.76630821829894,-4.82686416035968,11.9574988119276));
#7297=CARTESIAN_POINT('Ctrl Pts',(-10.3162203971305,-5.14105323712323,9.90313394764108));
#7298=CARTESIAN_POINT('Ctrl Pts',(-8.96397867699314,-4.45500100614754,10.2799584618669));
#7299=CARTESIAN_POINT('Ctrl Pts',(-9.1072016651553,-4.14741471865905,11.8063951598433));
#7300=CARTESIAN_POINT('Ctrl Pts',(-10.3599049752557,-4.76217486595153,9.84945417345977));
#7301=CARTESIAN_POINT('Ctrl Pts',(-9.11471603103977,-4.14482487528738,10.2890308821851));
#7302=CARTESIAN_POINT('Ctrl Pts',(-9.25650767056149,-3.80142989829907,11.6990353645558));
#7303=CARTESIAN_POINT('Ctrl Pts',(-10.4189001022453,-4.00398065568352,9.721683600557));
#7304=CARTESIAN_POINT('Ctrl Pts',(-9.3823816234562,-3.49904576722659,10.2437089713902));
#7305=CARTESIAN_POINT('Ctrl Pts',(-9.50950469399203,-3.11498392064292,11.4434912150781));
#7306=CARTESIAN_POINT('Ctrl Pts',(-10.4347636861683,-3.62198765253324,9.64735037171816));
#7307=CARTESIAN_POINT('Ctrl Pts',(-9.50257136926293,-3.16134167300405,10.1926151994274));
#7308=CARTESIAN_POINT('Ctrl Pts',(-9.61464424937305,-2.77202715941802,11.2948219712105));
#7309=CARTESIAN_POINT('Ctrl Pts',(-10.4418094540168,-2.85058636557395,9.48313222005232));
#7310=CARTESIAN_POINT('Ctrl Pts',(-9.70486490881434,-2.46757137018015,10.0437869313745));
#7311=CARTESIAN_POINT('Ctrl Pts',(-9.78671026371757,-2.08466339996095,10.9663778363833));
#7312=CARTESIAN_POINT('Ctrl Pts',(-10.4329171345597,-2.46024219210386,9.39296418997138));
#7313=CARTESIAN_POINT('Ctrl Pts',(-9.78912496618977,-2.10913674788569,9.94696884746788));
#7314=CARTESIAN_POINT('Ctrl Pts',(-9.85371162411618,-1.73943985085122,10.7860367058016));
#7315=CARTESIAN_POINT('Ctrl Pts',(-10.3710024490938,-1.28219336365977,9.10529667731764));
#7316=CARTESIAN_POINT('Ctrl Pts',(-9.97676127425813,-1.03561990945101,9.60995022839333));
#7317=CARTESIAN_POINT('Ctrl Pts',(-9.99941461087311,-0.704872753911718,
10.2106832300891));
#7318=CARTESIAN_POINT('Ctrl Pts',(-10.2846151359094,-0.506120192602798,
8.89580416339026));
#7319=CARTESIAN_POINT('Ctrl Pts',(-10.0255633361174,-0.29691220283424,9.32054117497725));
#7320=CARTESIAN_POINT('Ctrl Pts',(-10.0219463652807,-0.0328249135895384,
9.79168270706518));
#7321=CARTESIAN_POINT('Ctrl Pts',(-10.032396097053,1.04288661560029,8.45879148701088));
#7322=CARTESIAN_POINT('Ctrl Pts',(-9.95996217948876,1.15092964781065,8.69237184195042));
#7323=CARTESIAN_POINT('Ctrl Pts',(-9.93838086697549,1.29192649972561,8.91762214995515));
#7324=CARTESIAN_POINT('Ctrl Pts',(-9.8656723829824,1.81784246744332,8.23021899754132));
#7325=CARTESIAN_POINT('Ctrl Pts',(-9.84845494002237,1.88209883934655,8.34531059201747));
#7326=CARTESIAN_POINT('Ctrl Pts',(-9.83126409379134,1.94625595090589,8.4604474397326));
#7327=CARTESIAN_POINT('Ctrl Pts',(-9.65925826289068,2.58819045102525,8.));
#7328=CARTESIAN_POINT('Ctrl Pts',(-9.65925826289068,2.58819045102525,8.));
#7329=CARTESIAN_POINT('Ctrl Pts',(-9.65925826289068,2.58819045102525,8.));
#7330=CARTESIAN_POINT('Ctrl Pts',(-10.0423545251959,-6.56895087439983,10.));
#7331=CARTESIAN_POINT('Ctrl Pts',(-10.1408406688832,-6.17990680833961,10.));
#7332=CARTESIAN_POINT('Ctrl Pts',(-10.2162788692254,-5.79126062750106,9.97233221567646));
#7333=CARTESIAN_POINT('Ctrl Pts',(-10.3327502239336,-5.01321293394617,9.88673268190063));
#7334=CARTESIAN_POINT('Ctrl Pts',(-10.3736304459015,-4.62385215559531,9.82830572643859));
#7335=CARTESIAN_POINT('Ctrl Pts',(-10.4268830795136,-3.8438710354149,9.69155908354253));
#7336=CARTESIAN_POINT('Ctrl Pts',(-10.4391527105892,-3.45201704337316,9.61279798983037));
#7337=CARTESIAN_POINT('Ctrl Pts',(-10.4388601420181,-2.67621933636512,9.44350384379107));
#7338=CARTESIAN_POINT('Ctrl Pts',(-10.4264202812404,-2.29146269287581,9.35282484136955));
#7339=CARTESIAN_POINT('Ctrl Pts',(-10.3570673161662,-1.14440546669344,9.0687433666061));
#7340=CARTESIAN_POINT('Ctrl Pts',(-10.2684739953883,-0.389207488605518,
8.86354442007235));
#7341=CARTESIAN_POINT('Ctrl Pts',(-10.0809480410673,0.734026304274402,8.54552077981019));
#7342=CARTESIAN_POINT('Ctrl Pts',(-10.0092245223922,1.10680482587314,8.4377136379673));
#7343=CARTESIAN_POINT('Ctrl Pts',(-9.84777152533679,1.8495592796151,8.22004456397749));
#7344=CARTESIAN_POINT('Ctrl Pts',(-9.75762371352207,2.2210855915595,8.10971233033392));
#7345=CARTESIAN_POINT('Ctrl Pts',(-9.65925826289068,2.58819045102525,8.));
#7346=CARTESIAN_POINT('Origin',(-10.352761804101,-38.6370330515627,8.));
#7347=CARTESIAN_POINT('Origin',(-18.0801684144135,-36.5664806907425,8.));
#7348=CARTESIAN_POINT('Origin',(-7.72740661031254,2.0705523608202,8.));
#7349=CARTESIAN_POINT('Origin',(80.,0.,-28.));
#7350=CARTESIAN_POINT('Origin',(80.,-8.,-28.));
#7351=CARTESIAN_POINT('Origin',(80.,8.,-28.));
#7352=CARTESIAN_POINT('Origin',(0.,8.,-28.));
#7353=CARTESIAN_POINT('Origin',(54.,8.,-28.));
#7354=CARTESIAN_POINT('Origin',(23.0198096393687,-8.,-28.));
#7355=CARTESIAN_POINT('Origin',(54.,-8.,-28.));
#7356=CARTESIAN_POINT('Origin',(54.,8.,-23.));
#7357=CARTESIAN_POINT('Origin',(49.,8.,-23.));
#7358=CARTESIAN_POINT('Origin',(54.,-8.,-23.));
#7359=CARTESIAN_POINT('Origin',(49.,-8.,-23.));
#7360=CARTESIAN_POINT('Origin',(49.,8.,-10.));
#7361=CARTESIAN_POINT('Origin',(49.,8.,-12.));
#7362=CARTESIAN_POINT('Origin',(49.,-8.,30.));
#7363=CARTESIAN_POINT('Origin',(49.,-8.,-12.));
#7364=CARTESIAN_POINT('Origin',(45.,10.,-12.));
#7365=CARTESIAN_POINT('Origin',(45.,8.,-12.));
#7366=CARTESIAN_POINT('Origin',(45.,-8.,-12.));
#7367=CARTESIAN_POINT('Origin',(45.,8.,-12.));
#7368=CARTESIAN_POINT('Origin',(45.,8.,-8.));
#7369=CARTESIAN_POINT('Origin',(45.,-8.,-12.));
#7370=CARTESIAN_POINT('Origin',(45.,-8.,-8.));
#7371=CARTESIAN_POINT('Origin',(0.,8.,-8.));
#7372=CARTESIAN_POINT('Ctrl Pts',(0.,10.,-8.));
#7373=CARTESIAN_POINT('Ctrl Pts',(0.21283996478035,10.,-8.06144156707443));
#7374=CARTESIAN_POINT('Ctrl Pts',(0.4262133032106,9.99718006517799,-8.12303992303043));
#7375=CARTESIAN_POINT('Ctrl Pts',(0.63952603930531,9.99149862373395,-8.18448908348713));
#7376=CARTESIAN_POINT('Ctrl Pts',(0.806878166272437,9.98704131224235,-8.23269833667588));
#7377=CARTESIAN_POINT('Ctrl Pts',(0.974192987912469,9.98082375407732,-8.28081555193822));
#7378=CARTESIAN_POINT('Ctrl Pts',(1.14118650650328,9.97284817866079,-8.32869315474917));
#7379=CARTESIAN_POINT('Ctrl Pts',(1.41442329560585,9.95979844693199,-8.40703106015045));
#7380=CARTESIAN_POINT('Ctrl Pts',(1.68739639326401,9.94202171183076,-8.48489994346883));
#7381=CARTESIAN_POINT('Ctrl Pts',(1.96017979151534,9.91942459279275,-8.56202062209405));
#7382=CARTESIAN_POINT('Ctrl Pts',(2.06661525717798,9.91060757935695,-8.59211180577427));
#7383=CARTESIAN_POINT('Ctrl Pts',(2.17302164588681,9.90105623937531,-8.62208885095276));
#7384=CARTESIAN_POINT('Ctrl Pts',(2.2794025303324,9.89076326460884,-8.65193418212132));
#7385=CARTESIAN_POINT('Ctrl Pts',(2.30959079625838,9.887842372749,-8.66040354951436));
#7386=CARTESIAN_POINT('Ctrl Pts',(2.33977974216733,9.88486148480699,-8.66886307566744));
#7387=CARTESIAN_POINT('Ctrl Pts',(2.3699680394493,9.88182053327789,-8.67731195215625));
#7388=CARTESIAN_POINT('Ctrl Pts',(2.60220683799433,9.8584264702423,-8.74230922267101));
#7389=CARTESIAN_POINT('Ctrl Pts',(2.83459916520224,9.83150383039383,-8.80676897495569));
#7390=CARTESIAN_POINT('Ctrl Pts',(3.06684870944628,9.80084819296531,-8.87031999281874));
#7391=CARTESIAN_POINT('Ctrl Pts',(3.29289063466214,9.77101192643735,-8.93217240451646));
#7392=CARTESIAN_POINT('Ctrl Pts',(3.51879773119167,9.73763927964958,-8.99316350389003));
#7393=CARTESIAN_POINT('Ctrl Pts',(3.74430919491659,9.70058815615854,-9.05296006183168));
#7394=CARTESIAN_POINT('Ctrl Pts',(3.96164829554026,9.66487973706699,-9.11058963821226));
#7395=CARTESIAN_POINT('Ctrl Pts',(4.17862027427997,9.6257545265827,-9.16710931434817));
#7396=CARTESIAN_POINT('Ctrl Pts',(4.39499769774148,9.58313143643332,-9.22223551765105));
#7397=CARTESIAN_POINT('Ctrl Pts',(4.44640094103968,9.57300577249843,-9.23533145712178));
#7398=CARTESIAN_POINT('Ctrl Pts',(4.49777064455629,9.56268291649156,-9.24834883534915));
#7399=CARTESIAN_POINT('Ctrl Pts',(4.54910377883995,9.55216219113866,-9.26128401249424));
#7400=CARTESIAN_POINT('Ctrl Pts',(4.59670393277784,9.54240654006993,-9.27327853478306));
#7401=CARTESIAN_POINT('Ctrl Pts',(4.64432976534029,9.53246904754701,-9.28521680416131));
#7402=CARTESIAN_POINT('Ctrl Pts',(4.69198628933828,9.52234638104957,-9.29709733486223));
#7403=CARTESIAN_POINT('Ctrl Pts',(4.88268243400821,9.48184083610209,-9.34463692044747));
#7404=CARTESIAN_POINT('Ctrl Pts',(5.07273585349363,9.43855777060046,-9.39093663099496));
#7405=CARTESIAN_POINT('Ctrl Pts',(5.26204605452408,9.39237389696166,-9.43572635477248));
#7406=CARTESIAN_POINT('Ctrl Pts',(5.45135625555453,9.34619002332286,-9.48051607854999));
#7407=CARTESIAN_POINT('Ctrl Pts',(5.63992377103605,9.29710539175112,-9.52379633480365));
#7408=CARTESIAN_POINT('Ctrl Pts',(5.82761537190849,9.24496973141032,-9.56526367359599));
#7409=CARTESIAN_POINT('Ctrl Pts',(6.0017388658103,9.19660292494044,-9.60373336472639));
#7410=CARTESIAN_POINT('Ctrl Pts',(6.17530928602799,9.14557355400822,-9.64070509993831));
#7411=CARTESIAN_POINT('Ctrl Pts',(6.34849967657397,9.09158877785136,-9.67587155789363));
#7412=CARTESIAN_POINT('Ctrl Pts',(6.49227413063132,9.04677317523686,-9.70506508461134));
#7413=CARTESIAN_POINT('Ctrl Pts',(6.63578649863589,8.99992038455735,-9.7330140518619));
#7414=CARTESIAN_POINT('Ctrl Pts',(6.77913102959258,8.95084501649208,-9.75952238095208));
#7415=CARTESIAN_POINT('Ctrl Pts',(6.82705860123601,8.93443655498206,-9.76838550138743));
#7416=CARTESIAN_POINT('Ctrl Pts',(6.87489556090825,8.91780410736466,-9.77707420344914));
#7417=CARTESIAN_POINT('Ctrl Pts',(6.92267225370638,8.900932814949,-9.78558675592926));
#7418=CARTESIAN_POINT('Ctrl Pts',(7.02826208232899,8.8636460801317,-9.80440009157212));
#7419=CARTESIAN_POINT('Ctrl Pts',(7.13377131742087,8.82508785857041,-9.82237616418793));
#7420=CARTESIAN_POINT('Ctrl Pts',(7.23918103178142,8.78520631381303,-9.83939178290976));
#7421=CARTESIAN_POINT('Ctrl Pts',(7.33826960340199,8.74771636017827,-9.85538701982521));
#7422=CARTESIAN_POINT('Ctrl Pts',(7.43727103940148,8.7090565798954,-9.87053379453038));
#7423=CARTESIAN_POINT('Ctrl Pts',(7.53613923050785,8.66916680576892,-9.88470078228711));
#7424=CARTESIAN_POINT('Ctrl Pts',(7.62793946795173,8.63212869780502,-9.89785499119271));
#7425=CARTESIAN_POINT('Ctrl Pts',(7.71962524418919,8.59402984758295,-9.91016457273228));
#7426=CARTESIAN_POINT('Ctrl Pts',(7.81112455777423,8.55481220143714,-9.92149650701163));
#7427=CARTESIAN_POINT('Ctrl Pts',(7.83242071210478,8.54568442755471,-9.92413397621027));
#7428=CARTESIAN_POINT('Ctrl Pts',(7.85370659135147,8.53649601348149,-9.92671835540356));
#7429=CARTESIAN_POINT('Ctrl Pts',(7.87498095141589,8.52724616974222,-9.92924772122224));
#7430=CARTESIAN_POINT('Ctrl Pts',(7.90803474685888,8.51287476482515,-9.93317757575689));
#7431=CARTESIAN_POINT('Ctrl Pts',(7.94103969858764,8.49836474728666,-9.93697197572982));
#7432=CARTESIAN_POINT('Ctrl Pts',(7.97398093621393,8.48371800839878,-9.94062280955171));
#7433=CARTESIAN_POINT('Ctrl Pts',(8.10713921252213,8.42451153516385,-9.9553805652962));
#7434=CARTESIAN_POINT('Ctrl Pts',(8.23955047791889,8.36300313693741,-9.96789588233122));
#7435=CARTESIAN_POINT('Ctrl Pts',(8.37100368129355,8.29902072598766,-9.97758707535957));
#7436=CARTESIAN_POINT('Ctrl Pts',(8.5025158548848,8.23500961237769,-9.98728261587992));
#7437=CARTESIAN_POINT('Ctrl Pts',(8.63306909525044,8.16852221503888,-9.99415151076986));
#7438=CARTESIAN_POINT('Ctrl Pts',(8.76245266057622,8.09937778327323,-9.99755974503551));
#7439=CARTESIAN_POINT('Ctrl Pts',(8.82332527562265,8.0668465853048,-9.99916325728931));
#7440=CARTESIAN_POINT('Ctrl Pts',(8.88393898903987,8.03372712800054,-10.));
#7441=CARTESIAN_POINT('Ctrl Pts',(8.94427190999916,8.,-10.));
#7442=CARTESIAN_POINT('Origin',(23.0198096393687,-8.,-8.));
#7443=CARTESIAN_POINT('Origin',(23.0198096393687,-8.,-8.));
#7444=CARTESIAN_POINT('Ctrl Pts',(8.94427190999916,8.,-10.));
#7445=CARTESIAN_POINT('Ctrl Pts',(7.4535599249993,6.66666666666667,-10.));
#7446=CARTESIAN_POINT('Ctrl Pts',(7.4535599249993,6.66666666666667,-12.));
#7447=CARTESIAN_POINT('Ctrl Pts',(8.63559126581112,8.17255772523996,-10.));
#7448=CARTESIAN_POINT('Ctrl Pts',(7.28674859645865,6.85316740868464,-10.1119004423149));
#7449=CARTESIAN_POINT('Ctrl Pts',(7.1963453492561,6.95424130474946,-11.9999999936655));
#7450=CARTESIAN_POINT('Ctrl Pts',(8.3121131913303,8.33340210364555,-9.97809158727753));
#7451=CARTESIAN_POINT('Ctrl Pts',(7.0857578605764,7.06684700154838,-10.1930933295107));
#7452=CARTESIAN_POINT('Ctrl Pts',(6.92676099287817,7.22233683920652,-11.9561831730231));
#7453=CARTESIAN_POINT('Ctrl Pts',(7.63587535845283,8.63406215912108,-9.90314699084021));
#7454=CARTESIAN_POINT('Ctrl Pts',(6.62329565969844,7.50556561411578,-10.2799808570395));
#7455=CARTESIAN_POINT('Ctrl Pts',(6.36322946527443,7.7234369320712,-11.8062939832124));
#7456=CARTESIAN_POINT('Ctrl Pts',(7.2812158082226,8.77432121126777,-9.84946977287322));
#7457=CARTESIAN_POINT('Ctrl Pts',(6.36269523253062,7.73144033956278,-10.2890463036146));
#7458=CARTESIAN_POINT('Ctrl Pts',(6.0676798404454,7.95720201860455,-11.6989395444534));
#7459=CARTESIAN_POINT('Ctrl Pts',(6.5641300432471,9.02754593552104,-9.72170297362382));
#7460=CARTESIAN_POINT('Ctrl Pts',(5.80818652806631,8.15711407220398,-10.2437141637145));
#7461=CARTESIAN_POINT('Ctrl Pts',(5.47010836911268,8.37924322604346,-11.4434059485407));
#7462=CARTESIAN_POINT('Ctrl Pts',(6.19926100338533,9.14173876763111,-9.64737102026923));
#7463=CARTESIAN_POINT('Ctrl Pts',(5.51309261372975,8.36060703660556,-10.1926166741021));
#7464=CARTESIAN_POINT('Ctrl Pts',(5.16605083626499,8.56956461250842,-11.2947420399208));
#7465=CARTESIAN_POINT('Ctrl Pts',(5.45597212807415,9.34820332767296,-9.48315423310803));
#7466=CARTESIAN_POINT('Ctrl Pts',(4.89531257093376,8.73555834498249,-10.0437832244647));
#7467=CARTESIAN_POINT('Ctrl Pts',(4.54664343995125,8.91367221299836,-10.9663084668338));
#7468=CARTESIAN_POINT('Ctrl Pts',(5.0766289420487,9.44064538242793,-9.39298629553885));
#7469=CARTESIAN_POINT('Ctrl Pts',(4.57089679609006,8.90971222415245,-9.9469634911357));
#7470=CARTESIAN_POINT('Ctrl Pts',(4.23052411852774,9.06774230389022,-10.7859725905476));
#7471=CARTESIAN_POINT('Ctrl Pts',(3.92270247763147,9.68574985722747,-9.10531767774583));
#7472=CARTESIAN_POINT('Ctrl Pts',(3.58251566415662,9.36878975994216,-9.60994176359841));
#7473=CARTESIAN_POINT('Ctrl Pts',(3.26891873105192,9.47624976235846,-10.2106353565519));
#7474=CARTESIAN_POINT('Ctrl Pts',(3.1507174065752,9.80317350273003,-8.89582219816542));
#7475=CARTESIAN_POINT('Ctrl Pts',(2.88160777767504,9.6071140055565,-9.32053341119141));
#7476=CARTESIAN_POINT('Ctrl Pts',(2.62559783884422,9.67195583771219,-9.79164439618922));
#7477=CARTESIAN_POINT('Ctrl Pts',(1.5892186944781,9.96046757643772,-8.45880167110642));
#7478=CARTESIAN_POINT('Ctrl Pts',(1.46611730572651,9.91846933304019,-8.69236693608767));
#7479=CARTESIAN_POINT('Ctrl Pts',(1.32434891203353,9.93411262756739,-8.91760334235447));
#7480=CARTESIAN_POINT('Ctrl Pts',(0.797519998304341,10.,-8.23022404894487));
#7481=CARTESIAN_POINT('Ctrl Pts',(0.731001164897924,10.,-8.34530828179051));
#7482=CARTESIAN_POINT('Ctrl Pts',(0.664585080192849,10.,-8.46043776212959));
#7483=CARTESIAN_POINT('Ctrl Pts',(1.07753648825376E-35,10.,-8.));
#7484=CARTESIAN_POINT('Ctrl Pts',(1.07753648825376E-35,10.,-8.));
#7485=CARTESIAN_POINT('Ctrl Pts',(1.07753648825376E-35,10.,-8.));
#7486=CARTESIAN_POINT('Origin',(8.94427190999916,8.,-12.));
#7487=CARTESIAN_POINT('Origin',(23.0198096393687,-30.,-8.));
#7488=CARTESIAN_POINT('Origin',(1.76944146100923,-24.3059810077445,-8.));
#7489=CARTESIAN_POINT('Origin',(0.,0.,-12.));
#7490=CARTESIAN_POINT('Origin',(-10.0423545251959,-6.56895087439983,-12.));
#7491=CARTESIAN_POINT('Origin',(-2.62535519378845,-40.7075854123829,-8.));
#7492=CARTESIAN_POINT('Ctrl Pts',(-8.36862877395289,-5.47412573060034,-12.0001188722594));
#7493=CARTESIAN_POINT('Ctrl Pts',(-8.36852928825905,-5.47406065456325,-10.));
#7494=CARTESIAN_POINT('Ctrl Pts',(-10.0423545251959,-6.56895087439983,-10.));
#7495=CARTESIAN_POINT('Ctrl Pts',(-8.57983705192027,-5.1512387964459,-12.0001154444351));
#7496=CARTESIAN_POINT('Ctrl Pts',(-8.50550690521628,-5.2646728693275,-10.1119069073858));
#7497=CARTESIAN_POINT('Ctrl Pts',(-10.1291400589616,-6.22612704243147,-10.));
#7498=CARTESIAN_POINT('Ctrl Pts',(-8.76902620446576,-4.82144682478795,-11.9562940408389));
#7499=CARTESIAN_POINT('Ctrl Pts',(-8.65989255015849,-5.01523379072277,-10.1931054083213));
#7500=CARTESIAN_POINT('Ctrl Pts',(-10.200781511727,-5.87204162762333,-9.97809158727756));
#7501=CARTESIAN_POINT('Ctrl Pts',(-9.10720166492718,-4.14741471914895,-11.8063951574117));
#7502=CARTESIAN_POINT('Ctrl Pts',(-8.96398266446,-4.45499244724459,-10.2800009404067));
#7503=CARTESIAN_POINT('Ctrl Pts',(-10.3161735940769,-5.14102949167403,-9.90314699084018));
#7504=CARTESIAN_POINT('Ctrl Pts',(-9.25650767032995,-3.80142989885983,-11.6990353622533));
#7505=CARTESIAN_POINT('Ctrl Pts',(-9.11471988127295,-4.14481555522226,-10.2890691536593));
#7506=CARTESIAN_POINT('Ctrl Pts',(-10.3598607887893,-4.7621529586233,-9.84946977287314));
#7507=CARTESIAN_POINT('Ctrl Pts',(-9.50950469377493,-3.1149839212988,-11.4434912130292));
#7508=CARTESIAN_POINT('Ctrl Pts',(-9.38238492417113,-3.49903579951157,-10.2437401110933));
#7509=CARTESIAN_POINT('Ctrl Pts',(-10.4188616368525,-4.00396191724158,-9.72170297362389));
#7510=CARTESIAN_POINT('Ctrl Pts',(-9.61464424917777,-2.77202716009635,-11.2948219692898));
#7511=CARTESIAN_POINT('Ctrl Pts',(-9.50257422100183,-3.16133177106954,-10.1926432341521));
#7512=CARTESIAN_POINT('Ctrl Pts',(-10.4347283860805,-3.6219702086617,-9.64737102026915));
#7513=CARTESIAN_POINT('Ctrl Pts',(-9.78671026356967,-2.08466340065288,-10.9663778347164));
#7514=CARTESIAN_POINT('Ctrl Pts',(-9.70486691749541,-2.46756197702794,-10.0438095639491));
#7515=CARTESIAN_POINT('Ctrl Pts',(-10.4417805198947,-2.85057132732743,-9.48315423310812));
#7516=CARTESIAN_POINT('Ctrl Pts',(-9.85371162399755,-1.73943985153029,-10.7860367042605));
#7517=CARTESIAN_POINT('Ctrl Pts',(-9.78912652600938,-2.10912782389522,-9.94698910171766));
#7518=CARTESIAN_POINT('Ctrl Pts',(-10.4328914468443,-2.46022818257953,-9.39298629553918));
#7519=CARTESIAN_POINT('Ctrl Pts',(-9.9994146108298,-0.704872754544601,-10.2106832289395));
#7520=CARTESIAN_POINT('Ctrl Pts',(-9.97676179901941,-1.03561225412241,-9.60996413263565));
#7521=CARTESIAN_POINT('Ctrl Pts',(-10.3709860435543,-1.28218310284341,-9.10531767774516));
#7522=CARTESIAN_POINT('Ctrl Pts',(-10.0219463652877,-0.0328249141047754,
-9.79168270614615));
#7523=CARTESIAN_POINT('Ctrl Pts',(-10.0255632543393,-0.296906212413206,
-9.32055186205687));
#7524=CARTESIAN_POINT('Ctrl Pts',(-10.2846041364368,-0.506111309397711,
-8.89582219816607));
#7525=CARTESIAN_POINT('Ctrl Pts',(-9.93838086701884,1.29192649944193,-8.91762214950163));
#7526=CARTESIAN_POINT('Ctrl Pts',(-9.95996170279527,1.15093276255534,-8.69237681786647));
#7527=CARTESIAN_POINT('Ctrl Pts',(-10.0323929389604,1.04289132628966,-8.45880167110577));
#7528=CARTESIAN_POINT('Ctrl Pts',(-9.83126409382562,1.94625595077792,-8.4604474395028));
#7529=CARTESIAN_POINT('Ctrl Pts',(-9.84845456277914,1.88210024723749,-8.3453131186297));
#7530=CARTESIAN_POINT('Ctrl Pts',(-9.86567162729979,1.81784528768922,-8.23022404897214));
#7531=CARTESIAN_POINT('Ctrl Pts',(-9.65925826289068,2.58819045102525,-8.));
#7532=CARTESIAN_POINT('Ctrl Pts',(-9.65925826289068,2.58819045102525,-8.));
#7533=CARTESIAN_POINT('Ctrl Pts',(-9.65925826289068,2.58819045102525,-8.));
#7534=CARTESIAN_POINT('Ctrl Pts',(-9.65925826289068,2.58819045102525,-8.));
#7535=CARTESIAN_POINT('Ctrl Pts',(-9.71434529937461,2.3826028320288,-8.06144156712679));
#7536=CARTESIAN_POINT('Ctrl Pts',(-9.76684653524052,2.17577016080905,-8.12303992313113));
#7537=CARTESIAN_POINT('Ctrl Pts',(-9.81656808291557,1.96825541453737,-8.18448908363342));
#7538=CARTESIAN_POINT('Ctrl Pts',(-9.85557656828771,1.80545203606357,-8.23269833677755));
#7539=CARTESIAN_POINT('Ctrl Pts',(-9.89287513061151,1.64222910640599,-8.28081555199389));
#7540=CARTESIAN_POINT('Ctrl Pts',(-9.92839241932418,1.47886152331472,-8.32869315475884));
#7541=CARTESIAN_POINT('Ctrl Pts',(-9.9865062312563,1.21155753295729,-8.40703106014776));
#7542=CARTESIAN_POINT('Ctrl Pts',(-10.0399858601837,0.943284810476372,-8.48489994345202));
#7543=CARTESIAN_POINT('Ctrl Pts',(-10.0887602579555,0.673947716385416,-8.56202062206502));
#7544=CARTESIAN_POINT('Ctrl Pts',(-10.107791202562,0.568856940234897,-8.59211180575455));
#7545=CARTESIAN_POINT('Ctrl Pts',(-10.126105316523,0.463604192569669,-8.62208885094254));
#7546=CARTESIAN_POINT('Ctrl Pts',(-10.1436964653019,0.358184130924323,-8.65193418212102));
#7547=CARTESIAN_POINT('Ctrl Pts',(-10.148688398579,0.328268522773503,-8.66040354951402));
#7548=CARTESIAN_POINT('Ctrl Pts',(-10.1536225560833,0.298336729680905,-8.6688630756671));
#7549=CARTESIAN_POINT('Ctrl Pts',(-10.1584985287406,0.26839001751361,-8.67731195215595));
#7550=CARTESIAN_POINT('Ctrl Pts',(-10.1960094231454,0.0380097350912643,
-8.74230922266695));
#7551=CARTESIAN_POINT('Ctrl Pts',(-10.230151710219,-0.193432107512816,-8.80676897494775));
#7552=CARTESIAN_POINT('Ctrl Pts',(-10.2606512435707,-0.425702203233516,
-8.87031999280698));
#7553=CARTESIAN_POINT('Ctrl Pts',(-10.2903355784068,-0.651764130616837,
-8.93217240449971));
#7554=CARTESIAN_POINT('Ctrl Pts',(-10.3165691359871,-0.87861110605177,-8.99316350386837));
#7555=CARTESIAN_POINT('Ctrl Pts',(-10.3391471606142,-1.10602798937071,-9.05296006180536));
#7556=CARTESIAN_POINT('Ctrl Pts',(-10.3609069748836,-1.32520345863631,-9.11058963818087));
#7557=CARTESIAN_POINT('Ctrl Pts',(-10.3792714039689,-1.5449086460783,-9.16710931431195));
#7558=CARTESIAN_POINT('Ctrl Pts',(-10.3941032585197,-1.76494485509671,-9.22223551761038));
#7559=CARTESIAN_POINT('Ctrl Pts',(-10.3976267565664,-1.81721729007841,-9.23533145709489));
#7560=CARTESIAN_POINT('Ctrl Pts',(-10.4009511009633,-1.86950836518269,-9.24834883533589));
#7561=CARTESIAN_POINT('Ctrl Pts',(-10.4040748534343,-1.92181532947563,-9.26128401249444));
#7562=CARTESIAN_POINT('Ctrl Pts',(-10.4069714445036,-1.97031849579353,-9.27327853478326));
#7563=CARTESIAN_POINT('Ctrl Pts',(-10.4096990363332,-2.01889352978961,-9.28521680416154));
#7564=CARTESIAN_POINT('Ctrl Pts',(-10.4122557073664,-2.06754613598716,-9.29709733486248));
#7565=CARTESIAN_POINT('Ctrl Pts',(-10.4224861494618,-2.26222807356218,-9.34463692044782));
#7566=CARTESIAN_POINT('Ctrl Pts',(-10.4298673632025,-2.45700806149994,-9.39093663099528));
#7567=CARTESIAN_POINT('Ctrl Pts',(-10.4342542523557,-2.65182093992959,-9.43572635477272));
#7568=CARTESIAN_POINT('Ctrl Pts',(-10.4386411415088,-2.84663381835925,-9.48051607855016));
#7569=CARTESIAN_POINT('Ctrl Pts',(-10.4400338924942,-3.0414800890347,-9.5237963348037));
#7570=CARTESIAN_POINT('Ctrl Pts',(-10.4382528726121,-3.23626995552021,-9.56526367359598));
#7571=CARTESIAN_POINT('Ctrl Pts',(-10.4366006015294,-3.41697858590976,-9.6037333647265));
#7572=CARTESIAN_POINT('Ctrl Pts',(-10.4322333446654,-3.59784211053558,-9.64070509993859));
#7573=CARTESIAN_POINT('Ctrl Pts',(-10.424913026651,-3.77910346984486,-9.67587155789407));
#7574=CARTESIAN_POINT('Ctrl Pts',(-10.4188360455742,-3.92957805965298,-9.70506508461163));
#7575=CARTESIAN_POINT('Ctrl Pts',(-10.4107234590705,-4.08032675684369,-9.73301405186205));
#7576=CARTESIAN_POINT('Ctrl Pts',(-10.4004205882445,-4.2314885812519,-9.75952238095208));
#7577=CARTESIAN_POINT('Ctrl Pts',(-10.3969757998292,-4.28202988283323,-9.76838550138742));
#7578=CARTESIAN_POINT('Ctrl Pts',(-10.3932912053441,-4.33254163184186,-9.77707420344913));
#7579=CARTESIAN_POINT('Ctrl Pts',(-10.3893603062851,-4.38305698510292,-9.78558675592924));
#7580=CARTESIAN_POINT('Ctrl Pts',(-10.3806727447637,-4.49469944466476,-9.80440009157233));
#7581=CARTESIAN_POINT('Ctrl Pts',(-10.3707361622177,-4.60659314183877,-9.82237616418834));
#7582=CARTESIAN_POINT('Ctrl Pts',(-10.3594955897594,-4.7187332106141,-9.83939178291037));
#7583=CARTESIAN_POINT('Ctrl Pts',(-10.3489290848045,-4.82414853503473,-9.85538701982603));
#7584=CARTESIAN_POINT('Ctrl Pts',(-10.3372100617195,-4.92978246632457,-9.87053379453139));
#7585=CARTESIAN_POINT('Ctrl Pts',(-10.3242684694988,-5.035606038763,-9.88470078228827));
#7586=CARTESIAN_POINT('Ctrl Pts',(-10.3122520542547,-5.13386442670699,-9.89785499119407));
#7587=CARTESIAN_POINT('Ctrl Pts',(-10.2991814159282,-5.23228679391394,-9.91016457273381));
#7588=CARTESIAN_POINT('Ctrl Pts',(-10.2849818436389,-5.33081861772194,-9.92149650701328));
#7589=CARTESIAN_POINT('Ctrl Pts',(-10.2816769414382,-5.35375156490583,-9.92413397621134));
#7590=CARTESIAN_POINT('Ctrl Pts',(-10.2783108059237,-5.3766902819571,-9.92671835540409));
#7591=CARTESIAN_POINT('Ctrl Pts',(-10.2748823525246,-5.39963377150023,-9.92924772122223));
#7592=CARTESIAN_POINT('Ctrl Pts',(-10.2695555931287,-5.43528087947289,-9.93317757575688));
#7593=CARTESIAN_POINT('Ctrl Pts',(-10.2640823025385,-5.47091668362685,-9.93697197572981));
#7594=CARTESIAN_POINT('Ctrl Pts',(-10.2584604588427,-5.50652633077284,-9.9406228095517));
#7595=CARTESIAN_POINT('Ctrl Pts',(-10.2357352951814,-5.65047111172067,-9.95538056529732));
#7596=CARTESIAN_POINT('Ctrl Pts',(-10.2105933020697,-5.79429011756483,-9.96789588233314));
#7597=CARTESIAN_POINT('Ctrl Pts',(-10.1828136314758,-5.93782402816916,-9.9775870753618));
#7598=CARTESIAN_POINT('Ctrl Pts',(-10.1550214988549,-6.08142232843084,-9.98728261588294));
#7599=CARTESIAN_POINT('Ctrl Pts',(-10.1245892696446,-6.22473527971416,-9.9941515107729));
#7600=CARTESIAN_POINT('Ctrl Pts',(-10.0912878080822,-6.367606102781,-9.99755974503757));
#7601=CARTESIAN_POINT('Ctrl Pts',(-10.0756200759097,-6.43482422733345,-9.99916325729003));
#7602=CARTESIAN_POINT('Ctrl Pts',(-10.0593171201802,-6.50194452483541,-10.));
#7603=CARTESIAN_POINT('Ctrl Pts',(-10.0423545251959,-6.56895087439983,-10.));
#7604=CARTESIAN_POINT('Origin',(-7.72740661031254,2.0705523608202,-8.));
#7605=CARTESIAN_POINT('Origin',(0.,0.,-25.));
#7606=CARTESIAN_POINT('Origin',(0.,0.,25.));
#7607=CARTESIAN_POINT('Origin',(-10.352761804101,-38.6370330515627,-13.));
#7608=CARTESIAN_POINT('Origin',(-10.352761804101,-38.6370330515627,13.));
#7770=UNCERTAINTY_MEASURE_WITH_UNIT(LENGTH_MEASURE(0.01),#7784,
'DISTANCE_ACCURACY_VALUE',
'Maximum model space distance between geometric entities at asserted c
onnectivities');
#7773=UNCERTAINTY_MEASURE_WITH_UNIT(LENGTH_MEASURE(0.01),#7784,
'DISTANCE_ACCURACY_VALUE',
'Maximum model space distance between geometric entities at asserted c
onnectivities');
#7780=(
GEOMETRIC_REPRESENTATION_CONTEXT(3)
GLOBAL_UNCERTAINTY_ASSIGNED_CONTEXT((#7770))
GLOBAL_UNIT_ASSIGNED_CONTEXT((#7784,#7786,#7787))
REPRESENTATION_CONTEXT('','3D')
);
#7783=(
GEOMETRIC_REPRESENTATION_CONTEXT(3)
GLOBAL_UNCERTAINTY_ASSIGNED_CONTEXT((#7773))
GLOBAL_UNIT_ASSIGNED_CONTEXT((#7784,#7786,#7787))
REPRESENTATION_CONTEXT('','3D')
);
#7784=(
LENGTH_UNIT()
NAMED_UNIT(*)
SI_UNIT(.MILLI.,.METRE.)
);
#7786=(
NAMED_UNIT(*)
PLANE_ANGLE_UNIT()
SI_UNIT($,.RADIAN.)
);
#7787=(
NAMED_UNIT(*)
SI_UNIT($,.STERADIAN.)
SOLID_ANGLE_UNIT()
);
#7794=SHAPE_DEFINITION_REPRESENTATION(#7804,#7824);
#7804=PRODUCT_DEFINITION_SHAPE('',$,#7834);
#7824=SHAPE_REPRESENTATION('',(#4478),#7780);
#7827=PRODUCT_DEFINITION_CONTEXT('part definition',#7856,'design');
#7834=PRODUCT_DEFINITION('Lever','Lever',#7843,#7827);
#7843=PRODUCT_DEFINITION_FORMATION('',$,#7864);
#7856=APPLICATION_CONTEXT(
'Core Data for Automotive Mechanical Design Process');
#7857=PRODUCT_CONTEXT('part definition',#7856,'mechanical');
#7864=PRODUCT('Lever','Lever','Lever',(#7857));
#7868=PRESENTATION_STYLE_ASSIGNMENT((#7873));
#7873=SURFACE_STYLE_USAGE(.BOTH.,#7878);
#7878=SURFACE_SIDE_STYLE('',(#7883));
#7883=SURFACE_STYLE_FILL_AREA(#7888);
#7888=FILL_AREA_STYLE('Opaque(61,176,222)',(#7893));
#7893=FILL_AREA_STYLE_COLOUR('Opaque(61,176,222)',#7898);
#7898=COLOUR_RGB('Opaque(61,176,222)',0.23921568627451,0.690196078431373,
0.870588235294118);
ENDSEC;
END-ISO-10303-21;
